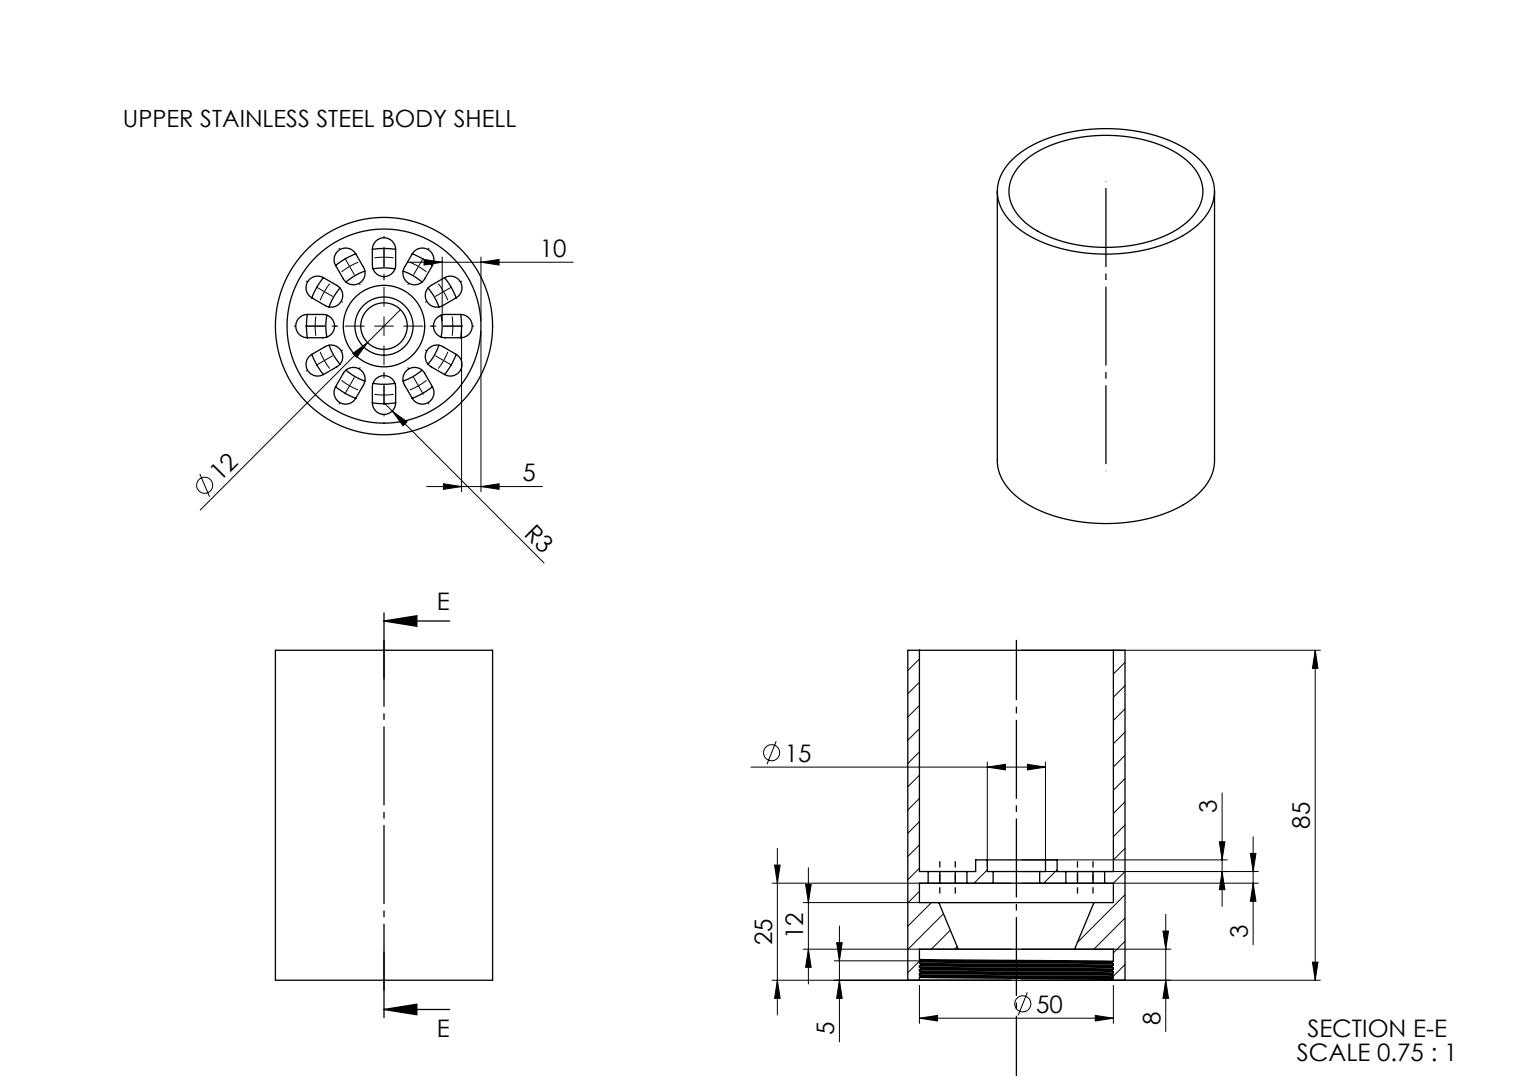
ISO-10303-21;
HEADER;
FILE_DESCRIPTION (('STEP AP214'),
    '1' );
FILE_NAME ('Upper Stainless Steel Body Shell.step',
    '2026-10-04T07:23:31',
    ( '' ),
    ( '' ),
    'SwSTEP 2.0',
    'SolidWorks 2026',
    '' );
FILE_SCHEMA (( 'AUTOMOTIVE_DESIGN' ));
ENDSEC;

DATA;
#1=ORIENTED_EDGE ( 'NONE', *, *, #1320, .F. ) ;
#4=ORIENTED_EDGE ( 'NONE', *, *, #9160, .T. ) ;
#5=AXIS2_PLACEMENT_3D ( 'NONE', #6946, #2717, #1088 ) ;
#6=DIRECTION ( 'NONE',  ( -0.000000000000000000, -1.000000000000000000, -0.000000000000000000 ) ) ;
#9=CARTESIAN_POINT ( 'NONE',  ( 1.507608415688466075E-15, 0.6437499990440845865, -24.62111388750000174 ) ) ;
#11=CARTESIAN_POINT ( 'NONE',  ( -18.60400172474273361, 25.00000000000000000, -7.276923788646512570 ) ) ;
#19=AXIS2_PLACEMENT_3D ( 'NONE', #2994, #5611, #7166 ) ;
#24=CIRCLE ( 'NONE', #8496, 7.500000000000000888 ) ;
#28=ADVANCED_FACE ( 'NONE', ( #7832 ), #3504, .F. ) ;
#29=( BOUNDED_CURVE ( )  B_SPLINE_CURVE ( 2, ( #1490, #9059, #4872, #2466, #7337, #5796, #6516, #4977, #5693, #9821, #8329, #10667, #710, #4147, #8268, #1536, #6469, #7289, #10712, #8217, #9874, #10767, #4922, #6628, #4037, #7506, #659, #2414, #7388, #6572, #5852, #9934, #4089, #2367, #5744, #10884, #9103, #7444, #3285, #9986, #9157, #6688, #4816, #10043, #9208, #3929, #1653, #8998, #5036, #8384, #2255, #5638, #1426, #9505, #8609, #7675, #9449, #6799, #7559, #10941, #4194, #1937, #2745, #104, #163, #6090, #1057, #8554, #946, #4431, #10334, #6920, #2627, #4366, #9319, #6026, #8495, #6851, #10273, #882, #2520 ),
 .UNSPECIFIED., .F., .F. ) 
 B_SPLINE_CURVE_WITH_KNOTS ( ( 3, 2, 2, 2, 2, 2, 2, 2, 2, 2, 2, 2, 2, 2, 2, 2, 2, 2, 2, 2, 2, 2, 2, 2, 2, 2, 2, 2, 2, 2, 2, 2, 2, 2, 2, 2, 2, 2, 2, 2, 3 ),
 ( 0.000000000000000000, 0.02500000000000000139, 0.05000000000000000278, 0.07499999999999999722, 0.1000000000000000056, 0.1250000000000000000, 0.1499999999999999944, 0.1749999999999999889, 0.2000000000000000111, 0.2250000000000000056, 0.2500000000000000000, 0.2750000000000000222, 0.2999999999999999889, 0.3250000000000000111, 0.3499999999999999778, 0.3750000000000000000, 0.4000000000000000222, 0.4249999999999999889, 0.4500000000000000111, 0.4749999999999999778, 0.5000000000000000000, 0.5250000000000000222, 0.5500000000000000444, 0.5749999999999999556, 0.5999999999999999778, 0.6250000000000000000, 0.6500000000000000222, 0.6750000000000000444, 0.6999999999999999556, 0.7249999999999999778, 0.7500000000000000000, 0.7750000000000000222, 0.8000000000000000444, 0.8249999999999999556, 0.8499999999999999778, 0.8750000000000000000, 0.9000000000000000222, 0.9250000000000000444, 0.9499999999999999556, 0.9749999999999999778, 1.000000000000000000 ),
 .UNSPECIFIED. ) 
 CURVE ( )  GEOMETRIC_REPRESENTATION_ITEM ( )  RATIONAL_B_SPLINE_CURVE ( ( 1.000000000000000000, 0.9238795325112867385, 1.000000000000000000, 0.9238795325112867385, 1.000000000000000000, 0.9238795325112867385, 1.000000000000000000, 0.9238795325112867385, 1.000000000000000000, 0.9238795325112867385, 1.000000000000000000, 0.9238795325112867385, 1.000000000000000000, 0.9238795325112867385, 1.000000000000000000, 0.9238795325112867385, 1.000000000000000000, 0.9238795325112867385, 1.000000000000000000, 0.9238795325112867385, 1.000000000000000000, 0.9238795325112867385, 1.000000000000000000, 0.9238795325112867385, 1.000000000000000000, 0.9238795325112867385, 1.000000000000000000, 0.9238795325112867385, 1.000000000000000000, 0.9238795325112867385, 1.000000000000000000, 0.9238795325112867385, 1.000000000000000000, 0.9238795325112867385, 1.000000000000000000, 0.9238795325112867385, 1.000000000000000000, 0.9238795325112867385, 1.000000000000000000, 0.9238795325112867385, 1.000000000000000000, 0.9238795325112867385, 1.000000000000000000, 0.9238795325112867385, 1.000000000000000000, 0.9238795325112867385, 1.000000000000000000, 0.9238795325112867385, 1.000000000000000000, 0.9238795325112867385, 1.000000000000000000, 0.9238795325112867385, 1.000000000000000000, 0.9238795325112867385, 1.000000000000000000, 0.9238795325112867385, 1.000000000000000000, 0.9238795325112867385, 1.000000000000000000, 0.9238795325112867385, 1.000000000000000000, 0.9238795325112867385, 1.000000000000000000, 0.9238795325112867385, 1.000000000000000000, 0.9238795325112867385, 1.000000000000000000, 0.9238795325112867385, 1.000000000000000000, 0.9238795325112867385, 1.000000000000000000, 0.9238795325112867385, 1.000000000000000000, 0.9238795325112867385, 1.000000000000000000, 0.9238795325112867385, 1.000000000000000000, 0.9238795325112867385, 1.000000000000000000, 0.9238795325112867385, 1.000000000000000000 ) ) 
 REPRESENTATION_ITEM ( '' )  );
#35=DIRECTION ( 'NONE',  ( 0.000000000000000000, 0.000000000000000000, 1.000000000000000000 ) ) ;
#36=FACE_OUTER_BOUND ( 'NONE', #8599, .T. ) ;
#38=FACE_OUTER_BOUND ( 'NONE', #4930, .T. ) ;
#40=CIRCLE ( 'NONE', #9387, 2.999999999999999112 ) ;
#46=DIRECTION ( 'NONE',  ( -0.000000000000000000, -1.000000000000000000, -0.000000000000000000 ) ) ;
#55=CARTESIAN_POINT ( 'NONE',  ( 15.13990010960488952, -0.001000000000001000089, -5.276923788646758595 ) ) ;
#56=CARTESIAN_POINT ( 'NONE',  ( 19.74999999999998934, -0.001000000000001000089, -3.000000000000067946 ) ) ;
#58=CARTESIAN_POINT ( 'NONE',  ( -2.999999999999998224, 25.00000000000000000, -15.75000000000000355 ) ) ;
#61=CARTESIAN_POINT ( 'NONE',  ( -4.592425496802574367E-15, 2.362499998088169129, 25.00000000000000000 ) ) ;
#64=VECTOR ( 'NONE', #5356, 1000.000000000000000 ) ;
#65=ORIENTED_EDGE ( 'NONE', *, *, #1287, .F. ) ;
#66=EDGE_CURVE ( 'NONE', #3225, #5856, #203, .T. ) ;
#68=ORIENTED_EDGE ( 'NONE', *, *, #3846, .T. ) ;
#71=DIRECTION ( 'NONE',  ( -0.000000000000000000, -1.000000000000000000, -0.000000000000000000 ) ) ;
#74=CARTESIAN_POINT ( 'NONE',  ( 24.62111388750000174, 2.393749999044084475, 0.000000000000000000 ) ) ;
#75=CARTESIAN_POINT ( 'NONE',  ( -25.00000000000000000, 0.4375000000000000000, -10.35533905932738108 ) ) ;
#76=CARTESIAN_POINT ( 'NONE',  ( 17.10400172474269098, 28.00000000000000000, 9.874999999999957367 ) ) ;
#84=ORIENTED_EDGE ( 'NONE', *, *, #2390, .T. ) ;
#86=DIRECTION ( 'NONE',  ( -0.000000000000000000, 1.000000000000000000, 0.000000000000000000 ) ) ;
#88=FACE_OUTER_BOUND ( 'NONE', #5727, .T. ) ;
#92=CARTESIAN_POINT ( 'NONE',  ( 12.47307621135333200, 25.00000000000000000, 15.60400172474264835 ) ) ;
#93=VERTEX_POINT ( 'NONE', #1861 ) ;
#95=DIRECTION ( 'NONE',  ( -0.000000000000000000, -1.000000000000000000, -0.000000000000000000 ) ) ;
#97=CARTESIAN_POINT ( 'NONE',  ( 24.99999999999999289, 5.549999998088169129, 10.35533905932739529 ) ) ;
#99=ORIENTED_EDGE ( 'NONE', *, *, #3561, .F. ) ;
#101=CARTESIAN_POINT ( 'NONE',  ( 17.10400172474269098, 28.00000000000000000, 9.874999999999957367 ) ) ;
#103=CARTESIAN_POINT ( 'NONE',  ( 19.74999999999998934, 25.00000000000000000, -3.000000000000067946 ) ) ;
#104=CARTESIAN_POINT ( 'NONE',  ( 24.62111388749999108, 4.156249999044084653, 10.19839929293507730 ) ) ;
#106=EDGE_CURVE ( 'NONE', #5745, #5240, #6492, .T. ) ;
#111=ORIENTED_EDGE ( 'NONE', *, *, #6802, .F. ) ;
#112=CARTESIAN_POINT ( 'NONE',  ( 3.061616997868383043E-15, 27.99999999999999645, 25.00000000000000000 ) ) ;
#117=CARTESIAN_POINT ( 'NONE',  ( 2.449293598294706513E-15, 20.00000000000000355, -20.00000000000000000 ) ) ;
#119=EDGE_CURVE ( 'NONE', #6443, #1427, #3381, .T. ) ;
#120=VERTEX_POINT ( 'NONE', #1095 ) ;
#121=ORIENTED_EDGE ( 'NONE', *, *, #10240, .T. ) ;
#122=VERTEX_POINT ( 'NONE', #5243 ) ;
#124=CARTESIAN_POINT ( 'NONE',  ( 0.000000000000000000, 85.00000000000000000, 0.000000000000000000 ) ) ;
#126=CARTESIAN_POINT ( 'NONE',  ( 17.67766952966369232, 0.7374999980881691286, -17.67766952966369232 ) ) ;
#127=CARTESIAN_POINT ( 'NONE',  ( 10.19839929293506486, 1.206249999044084698, 24.62111388749999819 ) ) ;
#128=CARTESIAN_POINT ( 'NONE',  ( -24.62111388750000884, 3.781249999044084653, 10.19839929293505421 ) ) ;
#129=CARTESIAN_POINT ( 'NONE',  ( -25.00000000000001066, 3.174999998088169573, 10.35533905932737397 ) ) ;
#130=EDGE_CURVE ( 'NONE', #7410, #4070, #2608, .T. ) ;
#132=LINE ( 'NONE', #3493, #145 ) ;
#133=FACE_BOUND ( 'NONE', #4065, .T. ) ;
#134=DIRECTION ( 'NONE',  ( 0.000000000000000000, 0.000000000000000000, -1.000000000000000000 ) ) ;
#138=CLOSED_SHELL ( 'NONE', ( #5912, #7027, #10918, #9263, #5268, #8033, #4039, #8931, #9209, #7081, #6514, #516, #6002, #10646, #9653, #6197, #4591, #507, #1397, #6646, #1299, #2039, #10092, #4594, #8749, #861, #6693, #7676, #7148, #10570, #5853, #5516, #7088, #717, #5052, #4023, #6869, #3689, #10249, #2799, #5302, #2691, #9344, #9035, #8964, #1267, #437, #3259, #9811, #1259, #7773, #2191, #3472, #3885, #1656, #6813, #3576, #3914, #8252, #9299, #6399, #2209, #4947, #674, #661, #4449, #10399, #4818, #868, #5935, #9573, #7951, #2937, #7004, #2676, #5317, #5105, #3750, #6202, #28, #5672, #1968, #3916, #4465, #4519, #8455, #4226, #4367, #4978, #6266, #8625, #8205, #7818, #6087, #10928, #4909, #2609 ) ) ;
#139=( BOUNDED_CURVE ( )  B_SPLINE_CURVE ( 2, ( #7817, #6880, #1965, #10238, #251, #129, #4337, #7756, #2653 ),
 .UNSPECIFIED., .F., .F. ) 
 B_SPLINE_CURVE_WITH_KNOTS ( ( 3, 2, 2, 2, 3 ),
 ( 0.4500000000000000111, 0.4749999999999999778, 0.5000000000000000000, 0.5250000000000000222, 0.5500000000000000444 ),
 .UNSPECIFIED. ) 
 CURVE ( )  GEOMETRIC_REPRESENTATION_ITEM ( )  RATIONAL_B_SPLINE_CURVE ( ( 1.000000000000000000, 0.9238795325112867385, 1.000000000000000000, 0.9238795325112867385, 1.000000000000000000, 0.9238795325112867385, 1.000000000000000000, 0.9238795325112867385, 1.000000000000000000 ) ) 
 REPRESENTATION_ITEM ( '' )  );
#140=ORIENTED_EDGE ( 'NONE', *, *, #5576, .T. ) ;
#141=ORIENTED_EDGE ( 'NONE', *, *, #3333, .T. ) ;
#145=VECTOR ( 'NONE', #2655, 1000.000000000000000 ) ;
#147=CARTESIAN_POINT ( 'NONE',  ( -17.10400172474254532, 28.00000000000000000, 9.875000000000202505 ) ) ;
#149=FACE_OUTER_BOUND ( 'NONE', #10908, .T. ) ;
#152=CARTESIAN_POINT ( 'NONE',  ( -24.62111388750000174, 3.893749999044084475, -3.015216831376932151E-15 ) ) ;
#155=ORIENTED_EDGE ( 'NONE', *, *, #4589, .F. ) ;
#156=CARTESIAN_POINT ( 'NONE',  ( 24.99999999999999289, 4.937500000000000888, 10.35533905932739529 ) ) ;
#157=CARTESIAN_POINT ( 'NONE',  ( 17.67766952966368521, 5.487499998088169129, 17.67766952966369232 ) ) ;
#163=CARTESIAN_POINT ( 'NONE',  ( 24.62111388750000174, 4.218749999044084653, 0.000000000000000000 ) ) ;
#168=ORIENTED_EDGE ( 'NONE', *, *, #8555, .T. ) ;
#169=DIRECTION ( 'NONE',  ( -0.000000000000000000, 1.000000000000000000, 0.000000000000000000 ) ) ;
#170=CARTESIAN_POINT ( 'NONE',  ( -17.10400172474254532, 28.00000000000000000, 9.875000000000202505 ) ) ;
#179=EDGE_LOOP ( 'NONE', ( #3319, #1358, #7705, #7107 ) ) ;
#181=ORIENTED_EDGE ( 'NONE', *, *, #2071, .F. ) ;
#186=CARTESIAN_POINT ( 'NONE',  ( -10.35533905932737575, 3.924999998088169129, -25.00000000000000000 ) ) ;
#187=CARTESIAN_POINT ( 'NONE',  ( -17.40975659021752975, 3.593749999044084653, -17.40975659021752975 ) ) ;
#188=FACE_OUTER_BOUND ( 'NONE', #7003, .T. ) ;
#189=AXIS2_PLACEMENT_3D ( 'NONE', #10549, #390, #1123 ) ;
#190=VECTOR ( 'NONE', #6922, 1000.000000000000000 ) ;
#192=PLANE ( 'NONE',  #1400 ) ;
#198=ORIENTED_EDGE ( 'NONE', *, *, #7378, .T. ) ;
#199=ORIENTED_EDGE ( 'NONE', *, *, #10771, .T. ) ;
#201=AXIS2_PLACEMENT_3D ( 'NONE', #9799, #474, #7991 ) ;
#203=LINE ( 'NONE', #6782, #2239 ) ;
#205=DIRECTION ( 'NONE',  ( -0.000000000000000000, 1.000000000000000000, -0.000000000000000000 ) ) ;
#208=CARTESIAN_POINT ( 'NONE',  ( -3.223142256880076948E-15, 28.00000000000000000, -15.75000000000000000 ) ) ;
#209=DIRECTION ( 'NONE',  ( 0.000000000000000000, 0.000000000000000000, 1.000000000000000000 ) ) ;
#210=CARTESIAN_POINT ( 'NONE',  ( 7.874999999999916511, 28.00000000000000000, -10.63990010960495702 ) ) ;
#211=CARTESIAN_POINT ( 'NONE',  ( 1.530808498934191521E-15, 1.250000000000000000, -25.00000000000000000 ) ) ;
#212=AXIS2_PLACEMENT_3D ( 'NONE', #8810, #4790, #575 ) ;
#214=ORIENTED_EDGE ( 'NONE', *, *, #10048, .F. ) ;
#215=DIRECTION ( 'NONE',  ( 0.000000000000000000, 0.000000000000000000, 1.000000000000000000 ) ) ;
#216=CARTESIAN_POINT ( 'NONE',  ( -10.35533905932739174, 4.299999998088169129, 24.99999999999999289 ) ) ;
#217=CIRCLE ( 'NONE', #6933, 25.00000000000000000 ) ;
#220=CARTESIAN_POINT ( 'NONE',  ( 3.061616997868383043E-15, 0.000000000000000000, 25.00000000000000000 ) ) ;
#225=AXIS2_PLACEMENT_3D ( 'NONE', #3856, #484, #9861 ) ;
#229=VECTOR ( 'NONE', #2900, 1000.000000000000000 ) ;
#230=CARTESIAN_POINT ( 'NONE',  ( 24.99999999999999289, 1.937500000000000000, 10.35533905932739529 ) ) ;
#231=CARTESIAN_POINT ( 'NONE',  ( -4.522825247065398226E-15, 4.968749999044083765, 24.62111388750000174 ) ) ;
#233=ORIENTED_EDGE ( 'NONE', *, *, #10324, .F. ) ;
#234=CARTESIAN_POINT ( 'NONE',  ( 1.530808498934191521E-15, 0.8624999980881691286, -25.00000000000000000 ) ) ;
#235=CARTESIAN_POINT ( 'NONE',  ( -17.67766952966368876, 2.375000000000000000, -17.67766952966369232 ) ) ;
#238=DIRECTION ( 'NONE',  ( -0.000000000000000000, 1.000000000000000000, -0.000000000000000000 ) ) ;
#239=VECTOR ( 'NONE', #5384, 1000.000000000000000 ) ;
#241=VERTEX_POINT ( 'NONE', #8761 ) ;
#247=EDGE_CURVE ( 'NONE', #3577, #5793, #9294, .T. ) ;
#248=CARTESIAN_POINT ( 'NONE',  ( -25.00000000000001421, 3.174999998088169129, 10.35533905932737397 ) ) ;
#249=CARTESIAN_POINT ( 'NONE',  ( -24.62111388750000174, 2.656249999044085097, -10.19839929293506131 ) ) ;
#251=CARTESIAN_POINT ( 'NONE',  ( -25.00000000000000000, 3.112499998088169129, -3.061616997868383043E-15 ) ) ;
#252=CYLINDRICAL_SURFACE ( 'NONE', #1418, 25.00000000000000000 ) ;
#255=CARTESIAN_POINT ( 'NONE',  ( -13.63990010960498367, 28.00000000000000000, -4.874999999999871214 ) ) ;
#258=VECTOR ( 'NONE', #8917, 1000.000000000000114 ) ;
#261=EDGE_CURVE ( 'NONE', #5968, #10806, #9690, .T. ) ;
#264=DIRECTION ( 'NONE',  ( 0.000000000000000000, 0.000000000000000000, 1.000000000000000000 ) ) ;
#269=CARTESIAN_POINT ( 'NONE',  ( -17.40975659021752975, 3.768749999044084475, -17.40975659021752975 ) ) ;
#284=CARTESIAN_POINT ( 'NONE',  ( 10.35533905932737930, 3.187500000000000444, -25.00000000000000000 ) ) ;
#285=CARTESIAN_POINT ( 'NONE',  ( -10.19839929293505776, 0.7062499990440845865, -24.62111388750000174 ) ) ;
#288=CARTESIAN_POINT ( 'NONE',  ( 1.530808498934191521E-15, 2.250000000000000444, -25.00000000000000000 ) ) ;
#297=DIRECTION ( 'NONE',  ( -2.168404344971010347E-16, 0.000000000000000000, -1.000000000000000000 ) ) ;
#298=CARTESIAN_POINT ( 'NONE',  ( 10.35533905932737930, 2.799999998088169573, -25.00000000000000000 ) ) ;
#299=CARTESIAN_POINT ( 'NONE',  ( 24.62111388749999463, 4.156249999044083765, 10.19839929293507730 ) ) ;
#300=CYLINDRICAL_SURFACE ( 'NONE', #10201, 2.999999999999997335 ) ;
#304=CARTESIAN_POINT ( 'NONE',  ( -15.75000000000000000, 25.00000000000000000, 1.681956355172181189E-13 ) ) ;
#305=ORIENTED_EDGE ( 'NONE', *, *, #6800, .T. ) ;
#306=ORIENTED_EDGE ( 'NONE', *, *, #2066, .F. ) ;
#311=LINE ( 'NONE', #7774, #4484 ) ;
#313=CARTESIAN_POINT ( 'NONE',  ( 0.000000000000000000, 0.000000000000000000, 0.000000000000000000 ) ) ;
#315=CYLINDRICAL_SURFACE ( 'NONE', #5866, 2.999999999999997335 ) ;
#316=CARTESIAN_POINT ( 'NONE',  ( 17.40975659021752975, 3.518749999044084920, -17.40975659021752975 ) ) ;
#321=ORIENTED_EDGE ( 'NONE', *, *, #1197, .F. ) ;
#323=EDGE_CURVE ( 'NONE', #8872, #4838, #1231, .T. ) ;
#326=FACE_OUTER_BOUND ( 'NONE', #1511, .T. ) ;
#329=CARTESIAN_POINT ( 'NONE',  ( -10.35533905932735621, 5.299999998088170905, 25.00000000000003197 ) ) ;
#331=AXIS2_PLACEMENT_3D ( 'NONE', #9569, #2055, #5387 ) ;
#333=ORIENTED_EDGE ( 'NONE', *, *, #7900, .F. ) ;
#335=EDGE_CURVE ( 'NONE', #6402, #2102, #10397, .T. ) ;
#339=LINE ( 'NONE', #8784, #5857 ) ;
#345=CARTESIAN_POINT ( 'NONE',  ( 2.999999999999999112, -0.001000000000001000089, 19.75000000000000000 ) ) ;
#350=CARTESIAN_POINT ( 'NONE',  ( -17.40975659021753330, 5.018749999044084475, 17.40975659021752975 ) ) ;
#351=CARTESIAN_POINT ( 'NONE',  ( 17.67766952966368521, 4.875000000000000000, 17.67766952966369232 ) ) ;
#360=ORIENTED_EDGE ( 'NONE', *, *, #10700, .T. ) ;
#368=CARTESIAN_POINT ( 'NONE',  ( 15.60400172474260927, -0.001000000000001000089, -12.47307621135339062 ) ) ;
#372=CIRCLE ( 'NONE', #6199, 2.999999999999999112 ) ;
#380=CYLINDRICAL_SURFACE ( 'NONE', #9214, 2.999999999999997335 ) ;
#389=AXIS2_PLACEMENT_3D ( 'NONE', #6634, #9992, #10835 ) ;
#390=DIRECTION ( 'NONE',  ( 0.000000000000000000, 0.000000000000000000, 1.000000000000000000 ) ) ;
#392=CARTESIAN_POINT ( 'NONE',  ( 15.60400172474269453, 25.00000000000000000, 12.47307621135327693 ) ) ;
#395=LINE ( 'NONE', #6422, #1735 ) ;
#398=EDGE_CURVE ( 'NONE', #963, #2292, #395, .T. ) ;
#400=EDGE_LOOP ( 'NONE', ( #8892, #7575 ) ) ;
#402=CIRCLE ( 'NONE', #9394, 2.999999999999999112 ) ;
#406=CARTESIAN_POINT ( 'NONE',  ( 24.62111388750000174, 2.393749999044084475, 0.000000000000000000 ) ) ;
#407=CARTESIAN_POINT ( 'NONE',  ( -25.00000000000000000, 3.437500000000000000, -10.35533905932738108 ) ) ;
#410=CARTESIAN_POINT ( 'NONE',  ( -17.67766952966368876, 0.9874999980881691286, -17.67766952966369232 ) ) ;
#412=AXIS2_PLACEMENT_3D ( 'NONE', #4846, #684, #4789 ) ;
#414=EDGE_CURVE ( 'NONE', #5784, #652, #8731, .T. ) ;
#416=VERTEX_POINT ( 'NONE', #5429 ) ;
#418=ORIENTED_EDGE ( 'NONE', *, *, #7281, .F. ) ;
#419=ORIENTED_EDGE ( 'NONE', *, *, #8806, .F. ) ;
#424=FACE_OUTER_BOUND ( 'NONE', #721, .T. ) ;
#433=DIRECTION ( 'NONE',  ( 1.000000000000000000, 0.000000000000000000, 0.000000000000000000 ) ) ;
#436=EDGE_CURVE ( 'NONE', #1816, #8189, #1374, .T. ) ;
#437=ADVANCED_FACE ( 'NONE', ( #450 ), #10554, .F. ) ;
#439=EDGE_CURVE ( 'NONE', #3209, #9663, #8791, .T. ) ;
#441=CARTESIAN_POINT ( 'NONE',  ( -4.592425496802574367E-15, 5.362499998088169129, 25.00000000000000000 ) ) ;
#442=CARTESIAN_POINT ( 'NONE',  ( 1.507608415688466075E-15, 2.643749999044084920, -24.62111388750000174 ) ) ;
#444=CARTESIAN_POINT ( 'NONE',  ( 24.62111388750000174, 5.218749999044084653, 0.000000000000000000 ) ) ;
#448=VERTEX_POINT ( 'NONE', #1591 ) ;
#450=FACE_OUTER_BOUND ( 'NONE', #4386, .T. ) ;
#451=PRODUCT ( 'Upper Stainless Steel Body Shell', 'Upper Stainless Steel Body Shell', '', ( #5141 ) ) ;
#452=ORIENTED_EDGE ( 'NONE', *, *, #7524, .T. ) ;
#456=CARTESIAN_POINT ( 'NONE',  ( -17.40975659021752975, 1.768749999044084475, -17.40975659021752975 ) ) ;
#458=CARTESIAN_POINT ( 'NONE',  ( -25.00000000000000000, 1.437500000000000000, -10.35533905932738108 ) ) ;
#459=EDGE_CURVE ( 'NONE', #2069, #3931, #29, .T. ) ;
#461=DIRECTION ( 'NONE',  ( 0.000000000000000000, -0.000000000000000000, 1.000000000000000000 ) ) ;
#463=CARTESIAN_POINT ( 'NONE',  ( 17.67766952966369232, 3.737499998088169573, -17.67766952966369232 ) ) ;
#464=ORIENTED_EDGE ( 'NONE', *, *, #335, .T. ) ;
#465=ORIENTED_EDGE ( 'NONE', *, *, #1592, .F. ) ;
#469=EDGE_CURVE ( 'NONE', #8735, #3294, #3407, .T. ) ;
#471=EDGE_LOOP ( 'NONE', ( #8532, #9181, #9575, #7189, #4997, #4095, #6051, #9424 ) ) ;
#474=DIRECTION ( 'NONE',  ( 0.000000000000000000, 1.000000000000000000, 0.000000000000000000 ) ) ;
#475=DIRECTION ( 'NONE',  ( 0.000000000000000000, 0.000000000000000000, 1.000000000000000000 ) ) ;
#476=ORIENTED_EDGE ( 'NONE', *, *, #10844, .F. ) ;
#483=DIRECTION ( 'NONE',  ( 0.000000000000000000, 1.000000000000000000, 0.000000000000000000 ) ) ;
#484=DIRECTION ( 'NONE',  ( -0.8660254037844451469, 0.000000000000000000, -0.4999999999999887312 ) ) ;
#486=VECTOR ( 'NONE', #920, 1000.000000000000000 ) ;
#489=CARTESIAN_POINT ( 'NONE',  ( 19.75000000000001066, 28.00000000000000000, 2.999999999999927613 ) ) ;
#493=DIRECTION ( 'NONE',  ( -0.000000000000000000, -1.000000000000000000, -0.000000000000000000 ) ) ;
#497=AXIS2_PLACEMENT_3D ( 'NONE', #5910, #6978, #9384 ) ;
#500=VERTEX_POINT ( 'NONE', #5316 ) ;
#504=CARTESIAN_POINT ( 'NONE',  ( 24.62111388749999463, 2.331249999044084031, 10.19839929293507730 ) ) ;
#506=CARTESIAN_POINT ( 'NONE',  ( 25.00000000000000000, 4.062500000000000000, -10.35533905932737753 ) ) ;
#507=ADVANCED_FACE ( 'NONE', ( #3586 ), #10212, .F. ) ;
#508=EDGE_CURVE ( 'NONE', #3100, #1857, #9259, .T. ) ;
#509=DIRECTION ( 'NONE',  ( -0.000000000000000000, -1.000000000000000000, -0.000000000000000000 ) ) ;
#510=CARTESIAN_POINT ( 'NONE',  ( 25.00000000000000000, 0.6749999980881690176, -10.35533905932737753 ) ) ;
#511=DIRECTION ( 'NONE',  ( 0.000000000000000000, 0.000000000000000000, 1.000000000000000000 ) ) ;
#513=ORIENTED_EDGE ( 'NONE', *, *, #1407, .T. ) ;
#516=ADVANCED_FACE ( 'NONE', ( #8437 ), #4251, .F. ) ;
#518=LINE ( 'NONE', #3202, #8425 ) ;
#520=EDGE_CURVE ( 'NONE', #5481, #3253, #2570, .T. ) ;
#522=DIRECTION ( 'NONE',  ( -0.000000000000000000, 1.000000000000000000, -0.000000000000000000 ) ) ;
#527=CIRCLE ( 'NONE', #8986, 2.999999999999998668 ) ;
#534=VECTOR ( 'NONE', #1707, 1000.000000000000000 ) ;
#538=EDGE_LOOP ( 'NONE', ( #10942, #1687, #7523, #476 ) ) ;
#539=VECTOR ( 'NONE', #2027, 1000.000000000000000 ) ;
#543=CARTESIAN_POINT ( 'NONE',  ( 10.19839929293505953, 3.581249999044085364, -24.62111388750000174 ) ) ;
#545=CARTESIAN_POINT ( 'NONE',  ( 19.75000000000000000, -0.001000000000001000089, -7.291468677852036884E-14 ) ) ;
#548=DIRECTION ( 'NONE',  ( -0.000000000000000000, 1.000000000000000000, -0.000000000000000000 ) ) ;
#551=VECTOR ( 'NONE', #10567, 1000.000000000000000 ) ;
#554=CARTESIAN_POINT ( 'NONE',  ( -24.62111388750000174, 3.893749999044084475, -3.015216831376932151E-15 ) ) ;
#555=CARTESIAN_POINT ( 'NONE',  ( -4.592425496802574367E-15, 4.750000000000000000, 25.00000000000000000 ) ) ;
#556=VECTOR ( 'NONE', #169, 1000.000000000000000 ) ;
#558=CARTESIAN_POINT ( 'NONE',  ( -13.63990010960481492, 28.00000000000000000, 7.875000000000163425 ) ) ;
#562=ORIENTED_EDGE ( 'NONE', *, *, #9891, .F. ) ;
#565=AXIS2_PLACEMENT_3D ( 'NONE', #8099, #5732, #433 ) ;
#571=( NAMED_UNIT ( * ) PLANE_ANGLE_UNIT ( ) SI_UNIT ( $, .RADIAN. ) );
#572=AXIS2_PLACEMENT_3D ( 'NONE', #5272, #10857, #4120 ) ;
#575=DIRECTION ( 'NONE',  ( 0.000000000000000000, 0.000000000000000000, -1.000000000000000000 ) ) ;
#577=CARTESIAN_POINT ( 'NONE',  ( -15.60400172474251690, 28.00000000000000000, 12.47307621135349720 ) ) ;
#580=ORIENTED_EDGE ( 'NONE', *, *, #5350, .F. ) ;
#582=EDGE_LOOP ( 'NONE', ( #4342, #8954, #2146, #5276, #930 ) ) ;
#584=ORIENTED_EDGE ( 'NONE', *, *, #5586, .F. ) ;
#598=LINE ( 'NONE', #3011, #2601 ) ;
#601=CARTESIAN_POINT ( 'NONE',  ( -24.62111388750000884, 2.956249999044084475, 10.19839929293505421 ) ) ;
#607=EDGE_LOOP ( 'NONE', ( #9268, #5348, #7147, #5082, #6374 ) ) ;
#608=ORIENTED_EDGE ( 'NONE', *, *, #5350, .T. ) ;
#611=CARTESIAN_POINT ( 'NONE',  ( 24.62111388750000174, 5.393749999044085364, 0.000000000000000000 ) ) ;
#612=EDGE_LOOP ( 'NONE', ( #729, #7297, #168, #8289 ) ) ;
#614=( BOUNDED_CURVE ( )  B_SPLINE_CURVE ( 2, ( #3089, #1344, #5599, #8078, #6437, #9838, #463, #1440, #10520 ),
 .UNSPECIFIED., .F., .F. ) 
 B_SPLINE_CURVE_WITH_KNOTS ( ( 3, 2, 2, 2, 3 ),
 ( 0.5500000000000000444, 0.5749999999999999556, 0.5999999999999999778, 0.6250000000000000000, 0.6500000000000000222 ),
 .UNSPECIFIED. ) 
 CURVE ( )  GEOMETRIC_REPRESENTATION_ITEM ( )  RATIONAL_B_SPLINE_CURVE ( ( 1.000000000000000000, 0.9238795325112867385, 1.000000000000000000, 0.9238795325112867385, 1.000000000000000000, 0.9238795325112867385, 1.000000000000000000, 0.9238795325112867385, 1.000000000000000000 ) ) 
 REPRESENTATION_ITEM ( '' )  );
#616=CARTESIAN_POINT ( 'NONE',  ( 25.00000000000000000, 1.674999998088169351, -10.35533905932737753 ) ) ;
#621=ORIENTED_EDGE ( 'NONE', *, *, #1452, .F. ) ;
#624=CARTESIAN_POINT ( 'NONE',  ( -10.19839929293505776, 0.5312499990440845421, -24.62111388750000174 ) ) ;
#633=ORIENTED_EDGE ( 'NONE', *, *, #8885, .F. ) ;
#634=VERTEX_POINT ( 'NONE', #10183 ) ;
#635=ORIENTED_EDGE ( 'NONE', *, *, #6976, .T. ) ;
#636=EDGE_CURVE ( 'NONE', #9541, #9951, #1793, .T. ) ;
#637=EDGE_LOOP ( 'NONE', ( #10358, #10252, #5332, #5163 ) ) ;
#640=CARTESIAN_POINT ( 'NONE',  ( -2.999999999999996447, 25.00000000000000000, 19.75000000000000000 ) ) ;
#641=EDGE_CURVE ( 'NONE', #2931, #7240, #5287, .T. ) ;
#642=CARTESIAN_POINT ( 'NONE',  ( 17.67766952966368521, 3.875000000000000000, 17.67766952966369232 ) ) ;
#644=CARTESIAN_POINT ( 'NONE',  ( -12.13990010960501031, -0.001000000000001000089, -10.47307621135320410 ) ) ;
#646=EDGE_CURVE ( 'NONE', #6058, #5812, #132, .T. ) ;
#651=CARTESIAN_POINT ( 'NONE',  ( 24.62111388750000174, 3.456249999044084920, -10.19839929293505776 ) ) ;
#652=VERTEX_POINT ( 'NONE', #1852 ) ;
#655=DIRECTION ( 'NONE',  ( -0.000000000000000000, -1.000000000000000000, -0.000000000000000000 ) ) ;
#659=CARTESIAN_POINT ( 'NONE',  ( -17.40975659021753330, 1.843749999044084653, 17.40975659021752975 ) ) ;
#661=ADVANCED_FACE ( 'NONE', ( #7154 ), #8753, .F. ) ;
#665=CARTESIAN_POINT ( 'NONE',  ( 10.19839929293506486, 1.031249999044084653, 24.62111388749999819 ) ) ;
#668=CARTESIAN_POINT ( 'NONE',  ( -7.875000000000116351, -0.001000000000001000089, -13.63990010960484334 ) ) ;
#669=LINE ( 'NONE', #7401, #7772 ) ;
#674=ADVANCED_FACE ( 'NONE', ( #2881 ), #5596, .F. ) ;
#675=CIRCLE ( 'NONE', #6169, 15.00000000000000178 ) ;
#678=ORIENTED_EDGE ( 'NONE', *, *, #6885, .F. ) ;
#679=ORIENTED_EDGE ( 'NONE', *, *, #641, .F. ) ;
#681=CARTESIAN_POINT ( 'NONE',  ( -4.522825247065398226E-15, 0.9687499990440845421, 24.62111388750000174 ) ) ;
#682=DIRECTION ( 'NONE',  ( 0.8660254037844399289, 0.000000000000000000, 0.4999999999999978351 ) ) ;
#683=CARTESIAN_POINT ( 'NONE',  ( -18.60400172474257730, 25.00000000000000000, 7.276923788646904256 ) ) ;
#684=DIRECTION ( 'NONE',  ( 0.000000000000000000, 1.000000000000000000, 0.000000000000000000 ) ) ;
#690=ORIENTED_EDGE ( 'NONE', *, *, #10232, .T. ) ;
#695=DIRECTION ( 'NONE',  ( 0.000000000000000000, 0.000000000000000000, -1.000000000000000000 ) ) ;
#696=AXIS2_PLACEMENT_3D ( 'NONE', #5366, #10629, #1398 ) ;
#697=VECTOR ( 'NONE', #9069, 1000.000000000000000 ) ;
#700=AXIS2_PLACEMENT_3D ( 'NONE', #7174, #7076, #7125 ) ;
#703=AXIS2_PLACEMENT_3D ( 'NONE', #3703, #2954, #6358 ) ;
#710=CARTESIAN_POINT ( 'NONE',  ( -4.522825247065398226E-15, 0.9687499990440845421, 24.62111388750000174 ) ) ;
#712=ORIENTED_EDGE ( 'NONE', *, *, #4302, .T. ) ;
#713=VECTOR ( 'NONE', #2272, 1000.000000000000000 ) ;
#714=ORIENTED_EDGE ( 'NONE', *, *, #5386, .T. ) ;
#715=ADVANCED_BREP_SHAPE_REPRESENTATION ( '', ( #10733, #7040 ), #6327 ) ;
#716=VERTEX_POINT ( 'NONE', #6382 ) ;
#717=ADVANCED_FACE ( 'NONE', ( #1386 ), #8129, .T. ) ;
#720=CARTESIAN_POINT ( 'NONE',  ( -10.19839929293505776, 3.531249999044084653, -24.62111388750000174 ) ) ;
#721=EDGE_LOOP ( 'NONE', ( #2374, #8932, #8644, #8469 ) ) ;
#722=CARTESIAN_POINT ( 'NONE',  ( 15.13990010960488952, 28.00000000000000000, -5.276923788646758595 ) ) ;
#728=VECTOR ( 'NONE', #9849, 1000.000000000000000 ) ;
#729=ORIENTED_EDGE ( 'NONE', *, *, #3055, .T. ) ;
#730=ORIENTED_EDGE ( 'NONE', *, *, #9628, .F. ) ;
#734=VECTOR ( 'NONE', #3164, 999.9999999999998863 ) ;
#735=CARTESIAN_POINT ( 'NONE',  ( 24.62111388749999463, 3.331249999044084920, 10.19839929293507730 ) ) ;
#736=DIRECTION ( 'NONE',  ( 0.000000000000000000, 0.000000000000000000, 1.000000000000000000 ) ) ;
#741=FACE_BOUND ( 'NONE', #6305, .T. ) ;
#745=ORIENTED_EDGE ( 'NONE', *, *, #6957, .T. ) ;
#746=CIRCLE ( 'NONE', #6240, 2.999999999999999112 ) ;
#750=EDGE_LOOP ( 'NONE', ( #8386, #3432 ) ) ;
#751=VECTOR ( 'NONE', #9383, 1000.000000000000000 ) ;
#752=VECTOR ( 'NONE', #4466, 1000.000000000000000 ) ;
#755=FACE_OUTER_BOUND ( 'NONE', #919, .T. ) ;
#767=ORIENTED_EDGE ( 'NONE', *, *, #8949, .F. ) ;
#778=EDGE_CURVE ( 'NONE', #2292, #917, #6434, .T. ) ;
#780=DIRECTION ( 'NONE',  ( -0.000000000000000000, 1.000000000000000000, -0.000000000000000000 ) ) ;
#781=CARTESIAN_POINT ( 'NONE',  ( 24.62111388750000174, 1.218749999044084431, 0.000000000000000000 ) ) ;
#783=ORIENTED_EDGE ( 'NONE', *, *, #7325, .T. ) ;
#788=LINE ( 'NONE', #4206, #9032 ) ;
#790=CARTESIAN_POINT ( 'NONE',  ( -12.47307621135311351, 28.00000000000000000, 15.60400172474282599 ) ) ;
#792=EDGE_CURVE ( 'NONE', #3303, #9988, #3484, .T. ) ;
#794=EDGE_LOOP ( 'NONE', ( #9614, #452, #10633, #7368 ) ) ;
#798=CARTESIAN_POINT ( 'NONE',  ( 24.62111388750000174, 3.393749999044084475, 0.000000000000000000 ) ) ;
#799=CARTESIAN_POINT ( 'NONE',  ( 17.40975659021752975, 1.343749999044084653, -17.40975659021752975 ) ) ;
#802=FACE_BOUND ( 'NONE', #1466, .T. ) ;
#803=DIRECTION ( 'NONE',  ( -0.4999999999999886757, 0.000000000000000000, 0.8660254037844452579 ) ) ;
#807=ORIENTED_EDGE ( 'NONE', *, *, #2469, .F. ) ;
#809=ORIENTED_EDGE ( 'NONE', *, *, #4102, .F. ) ;
#814=DIRECTION ( 'NONE',  ( 0.8660254037844344888, 0.000000000000000000, -0.5000000000000074385 ) ) ;
#815=CARTESIAN_POINT ( 'NONE',  ( 0.000000000000000000, 85.00000000000000000, -25.00000000000000000 ) ) ;
#822=CYLINDRICAL_SURFACE ( 'NONE', #4192, 5.999999999999999112 ) ;
#831=DIRECTION ( 'NONE',  ( -3.469446951953617344E-15, 0.000000000000000000, 1.000000000000000000 ) ) ;
#832=CARTESIAN_POINT ( 'NONE',  ( -17.40975659021753330, 0.8437499990440846531, 17.40975659021752975 ) ) ;
#833=FACE_OUTER_BOUND ( 'NONE', #9928, .T. ) ;
#835=DIRECTION ( 'NONE',  ( 0.000000000000000000, 1.000000000000000000, -0.000000000000000000 ) ) ;
#837=CARTESIAN_POINT ( 'NONE',  ( -15.75000000000003553, -0.001000000000001000089, -2.999999999999832578 ) ) ;
#841=ORIENTED_EDGE ( 'NONE', *, *, #5114, .F. ) ;
#843=LINE ( 'NONE', #1077, #3128 ) ;
#846=CARTESIAN_POINT ( 'NONE',  ( -24.62111388750000174, 1.893749999044084475, -3.015216831376932151E-15 ) ) ;
#847=CARTESIAN_POINT ( 'NONE',  ( 17.40975659021752620, 2.093749999044084653, 17.40975659021753330 ) ) ;
#848=VECTOR ( 'NONE', #6164, 1000.000000000000000 ) ;
#849=VERTEX_POINT ( 'NONE', #3356 ) ;
#852=VECTOR ( 'NONE', #9676, 1000.000000000000000 ) ;
#855=EDGE_CURVE ( 'NONE', #3253, #7713, #7400, .T. ) ;
#857=VERTEX_POINT ( 'NONE', #5867 ) ;
#861=ADVANCED_FACE ( 'NONE', ( #10783 ), #9999, .F. ) ;
#864=CARTESIAN_POINT ( 'NONE',  ( 10.47307621135333200, -0.001000000000001000089, 12.13990010960489840 ) ) ;
#867=DIRECTION ( 'NONE',  ( -0.000000000000000000, -1.000000000000000000, -0.000000000000000000 ) ) ;
#868=ADVANCED_FACE ( 'NONE', ( #9887 ), #9068, .F. ) ;
#876=PLANE ( 'NONE',  #6905 ) ;
#879=AXIS2_PLACEMENT_3D ( 'NONE', #8342, #7460, #2375 ) ;
#881=DIRECTION ( 'NONE',  ( 0.000000000000000000, 1.000000000000000000, 0.000000000000000000 ) ) ;
#882=CARTESIAN_POINT ( 'NONE',  ( 24.62111388749999108, 5.156249999044084653, 10.19839929293507730 ) ) ;
#883=VERTEX_POINT ( 'NONE', #5047 ) ;
#884=AXIS2_PLACEMENT_3D ( 'NONE', #2622, #6916, #2566 ) ;
#888=DIRECTION ( 'NONE',  ( -0.000000000000000000, -1.000000000000000000, -0.000000000000000000 ) ) ;
#890=DIRECTION ( 'NONE',  ( -0.5000000000000073275, 0.000000000000000000, -0.8660254037844343777 ) ) ;
#891=ORIENTED_EDGE ( 'NONE', *, *, #4982, .F. ) ;
#892=DIRECTION ( 'NONE',  ( -1.734723475976808672E-15, 0.000000000000000000, 1.000000000000000000 ) ) ;
#896=DIRECTION ( 'NONE',  ( -0.000000000000000000, -1.000000000000000000, -0.000000000000000000 ) ) ;
#900=ORIENTED_EDGE ( 'NONE', *, *, #1135, .T. ) ;
#901=EDGE_LOOP ( 'NONE', ( #712, #6645, #5603, #3659 ) ) ;
#902=ORIENTED_EDGE ( 'NONE', *, *, #7656, .F. ) ;
#905=LINE ( 'NONE', #10177, #2160 ) ;
#906=CARTESIAN_POINT ( 'NONE',  ( -24.62111388750000174, 1.831249999044084475, -10.19839929293506131 ) ) ;
#907=CARTESIAN_POINT ( 'NONE',  ( 24.99999999999999289, 0.9374999999999998890, 10.35533905932739529 ) ) ;
#916=EDGE_CURVE ( 'NONE', #4798, #3364, #4990, .T. ) ;
#917=VERTEX_POINT ( 'NONE', #7517 ) ;
#918=AXIS2_PLACEMENT_3D ( 'NONE', #5764, #9129, #6604 ) ;
#919=EDGE_LOOP ( 'NONE', ( #68, #2381, #5556, #7537 ) ) ;
#920=DIRECTION ( 'NONE',  ( 0.000000000000000000, 1.000000000000000000, -0.000000000000000000 ) ) ;
#921=EDGE_CURVE ( 'NONE', #8104, #9229, #2426, .T. ) ;
#923=ORIENTED_EDGE ( 'NONE', *, *, #1153, .F. ) ;
#927=DIRECTION ( 'NONE',  ( -0.8660254037844402619, -0.4999999999999971134, 0.000000000000000000 ) ) ;
#928=DIRECTION ( 'NONE',  ( -0.000000000000000000, 1.000000000000000000, -0.000000000000000000 ) ) ;
#930=ORIENTED_EDGE ( 'NONE', *, *, #5640, .F. ) ;
#931=EDGE_CURVE ( 'NONE', #3835, #5793, #3995, .T. ) ;
#932=AXIS2_PLACEMENT_3D ( 'NONE', #8431, #1760, #6794 ) ;
#933=CIRCLE ( 'NONE', #6057, 2.999999999999997335 ) ;
#935=VECTOR ( 'NONE', #8204, 1000.000000000000000 ) ;
#936=EDGE_CURVE ( 'NONE', #10359, #5295, #2788, .T. ) ;
#939=DIRECTION ( 'NONE',  ( 0.000000000000000000, 0.000000000000000000, 1.000000000000000000 ) ) ;
#940=AXIS2_PLACEMENT_3D ( 'NONE', #6069, #10195, #10363 ) ;
#941=CARTESIAN_POINT ( 'NONE',  ( -15.60400172474278158, 28.00000000000000000, -12.47307621135316680 ) ) ;
#946=CARTESIAN_POINT ( 'NONE',  ( 1.507608415688466075E-15, 4.468749999044084653, -24.62111388750000174 ) ) ;
#952=CARTESIAN_POINT ( 'NONE',  ( 17.67766952966368521, 1.875000000000000000, 17.67766952966369232 ) ) ;
#953=AXIS2_PLACEMENT_3D ( 'NONE', #6193, #7077, #10436 ) ;
#954=CARTESIAN_POINT ( 'NONE',  ( 10.19839929293506486, 5.031249999044083765, 24.62111388749999819 ) ) ;
#961=CARTESIAN_POINT ( 'NONE',  ( 0.000000000000000000, 28.00000000000000000, -7.500000000000000888 ) ) ;
#963=VERTEX_POINT ( 'NONE', #10056 ) ;
#965=EDGE_LOOP ( 'NONE', ( #9121, #8922, #199, #5165 ) ) ;
#966=ORIENTED_EDGE ( 'NONE', *, *, #8610, .T. ) ;
#968=CARTESIAN_POINT ( 'NONE',  ( 3.957930336368489021E-15, 28.00000000000000000, 19.75000000000000000 ) ) ;
#970=CARTESIAN_POINT ( 'NONE',  ( 1.507608415688466075E-15, 0.6437499990440845865, -24.62111388750000174 ) ) ;
#971=CARTESIAN_POINT ( 'NONE',  ( 17.40975659021752620, 1.268749999044084475, 17.40975659021753330 ) ) ;
#972=CARTESIAN_POINT ( 'NONE',  ( -24.62111388750000884, 2.781249999044085541, 10.19839929293505421 ) ) ;
#974=FACE_BOUND ( 'NONE', #8390, .T. ) ;
#975=CYLINDRICAL_SURFACE ( 'NONE', #2480, 25.00000000000000000 ) ;
#976=LINE ( 'NONE', #2030, #752 ) ;
#980=DIRECTION ( 'NONE',  ( 0.000000000000000000, -1.000000000000000000, 0.000000000000000000 ) ) ;
#981=ORIENTED_EDGE ( 'NONE', *, *, #5799, .F. ) ;
#983=CARTESIAN_POINT ( 'NONE',  ( 0.000000000000000000, 20.00000000000000355, 20.00000000000000000 ) ) ;
#989=ORIENTED_EDGE ( 'NONE', *, *, #1979, .F. ) ;
#993=CARTESIAN_POINT ( 'NONE',  ( -10.35533905932737575, 3.924999998088168685, -25.00000000000000000 ) ) ;
#994=EDGE_CURVE ( 'NONE', #9664, #5784, #7058, .T. ) ;
#998=DIRECTION ( 'NONE',  ( 0.5000000000000009992, 0.000000000000000000, 0.8660254037844380415 ) ) ;
#1005=CARTESIAN_POINT ( 'NONE',  ( 25.00000000000000000, 3.062500000000000000, -10.35533905932737753 ) ) ;
#1006=DIRECTION ( 'NONE',  ( 0.000000000000000000, 1.000000000000000000, 0.000000000000000000 ) ) ;
#1009=DIRECTION ( 'NONE',  ( -0.8660254037844328234, 0.000000000000000000, 0.5000000000000098810 ) ) ;
#1011=DIRECTION ( 'NONE',  ( -0.4999999999999888978, 0.000000000000000000, 0.8660254037844450359 ) ) ;
#1012=FACE_BOUND ( 'NONE', #6871, .T. ) ;
#1014=DIRECTION ( 'NONE',  ( -0.000000000000000000, 1.000000000000000000, -0.000000000000000000 ) ) ;
#1018=EDGE_LOOP ( 'NONE', ( #3836, #1523 ) ) ;
#1020=CARTESIAN_POINT ( 'NONE',  ( 9.184850993605149917E-16, 31.00000000000000000, 7.500000000000000888 ) ) ;
#1023=CARTESIAN_POINT ( 'NONE',  ( 17.67766952966369232, 4.737499998088169129, -17.67766952966369232 ) ) ;
#1024=CARTESIAN_POINT ( 'NONE',  ( -17.40975659021753330, 4.843749999044083765, 17.40975659021752975 ) ) ;
#1028=FACE_OUTER_BOUND ( 'NONE', #4958, .T. ) ;
#1029=STYLED_ITEM ( 'NONE', ( #4490 ), #10733 ) ;
#1033=EDGE_LOOP ( 'NONE', ( #9297, #6954, #9499, #8643 ) ) ;
#1034=ORIENTED_EDGE ( 'NONE', *, *, #10874, .F. ) ;
#1036=( GEOMETRIC_REPRESENTATION_CONTEXT ( 3 ) GLOBAL_UNCERTAINTY_ASSIGNED_CONTEXT ( ( #3144 ) ) GLOBAL_UNIT_ASSIGNED_CONTEXT ( ( #2061, #10617, #3724 ) ) REPRESENTATION_CONTEXT ( 'NONE', 'WORKASPACE' ) );
#1038=PLANE ( 'NONE',  #2001 ) ;
#1040=DIRECTION ( 'NONE',  ( -0.000000000000000000, -1.000000000000000000, -0.000000000000000000 ) ) ;
#1042=CARTESIAN_POINT ( 'NONE',  ( -7.875000000000116351, 25.00000000000000000, -13.63990010960484334 ) ) ;
#1044=FACE_OUTER_BOUND ( 'NONE', #8271, .T. ) ;
#1046=APPLICATION_CONTEXT ( 'automotive_design' ) ;
#1050=CARTESIAN_POINT ( 'NONE',  ( -4.592425496802574367E-15, 5.362499998088169129, 25.00000000000000000 ) ) ;
#1052=( BOUNDED_CURVE ( )  B_SPLINE_CURVE ( 2, ( #2193, #5570, #7270, #10650, #3059, #6455, #2236, #1412, #4073 ),
 .UNSPECIFIED., .F., .F. ) 
 B_SPLINE_CURVE_WITH_KNOTS ( ( 3, 2, 2, 2, 3 ),
 ( 0.7500000000000000000, 0.7750000000000000222, 0.8000000000000000444, 0.8250000000000000666, 0.8500000000000000888 ),
 .UNSPECIFIED. ) 
 CURVE ( )  GEOMETRIC_REPRESENTATION_ITEM ( )  RATIONAL_B_SPLINE_CURVE ( ( 1.000000000000000000, 0.9238795325112867385, 1.000000000000000000, 0.9238795325112867385, 1.000000000000000000, 0.9238795325112867385, 1.000000000000000000, 0.9238795325112864054, 1.000000000000000444 ) ) 
 REPRESENTATION_ITEM ( '' )  );
#1053=LINE ( 'NONE', #4308, #3154 ) ;
#1057=CARTESIAN_POINT ( 'NONE',  ( 17.40975659021752975, 4.343749999044084653, -17.40975659021752975 ) ) ;
#1064=VERTEX_POINT ( 'NONE', #4444 ) ;
#1065=FACE_OUTER_BOUND ( 'NONE', #3101, .T. ) ;
#1066=EDGE_CURVE ( 'NONE', #241, #6044, #675, .T. ) ;
#1075=EDGE_CURVE ( 'NONE', #9988, #3378, #10729, .T. ) ;
#1076=ORIENTED_EDGE ( 'NONE', *, *, #4297, .F. ) ;
#1077=CARTESIAN_POINT ( 'NONE',  ( -15.74999999999997158, -0.001000000000001000089, 3.000000000000165645 ) ) ;
#1080=CARTESIAN_POINT ( 'NONE',  ( -25.00000000000001421, 4.174999998088169129, 10.35533905932737397 ) ) ;
#1081=CARTESIAN_POINT ( 'NONE',  ( -24.62111388750000884, 4.781249999044083765, 10.19839929293505421 ) ) ;
#1086=DIRECTION ( 'NONE',  ( 0.000000000000000000, -1.000000000000000000, 0.000000000000000000 ) ) ;
#1087=LINE ( 'NONE', #7821, #4265 ) ;
#1088=DIRECTION ( 'NONE',  ( 0.000000000000000000, 0.000000000000000000, 1.000000000000000000 ) ) ;
#1095=CARTESIAN_POINT ( 'NONE',  ( 2.999999999999997335, 28.00000000000000000, -15.75000000000000355 ) ) ;
#1098=CARTESIAN_POINT ( 'NONE',  ( -4.592425496802574367E-15, 2.750000000000000000, 25.00000000000000000 ) ) ;
#1099=FACE_OUTER_BOUND ( 'NONE', #4676, .T. ) ;
#1100=DIRECTION ( 'NONE',  ( -0.000000000000000000, -1.000000000000000000, -0.000000000000000000 ) ) ;
#1103=CARTESIAN_POINT ( 'NONE',  ( 24.62111388749999463, 4.331249999044084475, 10.19839929293507730 ) ) ;
#1106=ORIENTED_EDGE ( 'NONE', *, *, #4297, .T. ) ;
#1114=CARTESIAN_POINT ( 'NONE',  ( 0.000000000000000000, 85.00000000000000000, -25.00000000000000000 ) ) ;
#1118=AXIS2_PLACEMENT_3D ( 'NONE', #8201, #3910, #5621 ) ;
#1119=FACE_OUTER_BOUND ( 'NONE', #5894, .T. ) ;
#1121=DIRECTION ( 'NONE',  ( 0.000000000000000000, 1.000000000000000000, -0.000000000000000000 ) ) ;
#1123=DIRECTION ( 'NONE',  ( 1.000000000000000000, 0.000000000000000000, -0.000000000000000000 ) ) ;
#1130=ORIENTED_EDGE ( 'NONE', *, *, #1287, .T. ) ;
#1131=CIRCLE ( 'NONE', #9596, 25.00000000000000000 ) ;
#1132=ORIENTED_EDGE ( 'NONE', *, *, #9956, .T. ) ;
#1135=EDGE_CURVE ( 'NONE', #6439, #7005, #598, .T. ) ;
#1139=CARTESIAN_POINT ( 'NONE',  ( 25.00000000000000000, 0.6749999980881691286, -10.35533905932737753 ) ) ;
#1140=CARTESIAN_POINT ( 'NONE',  ( 10.35533905932738286, 3.424999998088169573, 24.99999999999999645 ) ) ;
#1142=CARTESIAN_POINT ( 'NONE',  ( 24.62111388750000174, 4.218749999044084653, 0.000000000000000000 ) ) ;
#1144=EDGE_CURVE ( 'NONE', #4659, #9481, #7929, .T. ) ;
#1150=AXIS2_PLACEMENT_3D ( 'NONE', #9805, #4699, #8881 ) ;
#1152=DIRECTION ( 'NONE',  ( 0.000000000000000000, 0.000000000000000000, -1.000000000000000000 ) ) ;
#1153=EDGE_CURVE ( 'NONE', #7275, #5714, #1385, .T. ) ;
#1157=EDGE_CURVE ( 'NONE', #7830, #2468, #8435, .T. ) ;
#1162=CARTESIAN_POINT ( 'NONE',  ( -25.00000000000000000, 1.500000000000000000, -3.061616997868383043E-15 ) ) ;
#1163=DIRECTION ( 'NONE',  ( 0.000000000000000000, 0.000000000000000000, 1.000000000000000000 ) ) ;
#1165=ORIENTED_EDGE ( 'NONE', *, *, #6990, .F. ) ;
#1170=DIRECTION ( 'NONE',  ( -0.000000000000000000, -1.000000000000000000, -0.000000000000000000 ) ) ;
#1173=ORIENTED_EDGE ( 'NONE', *, *, #4852, .F. ) ;
#1180=CARTESIAN_POINT ( 'NONE',  ( 0.000000000000000000, 85.00000000000000000, -28.00000000000000000 ) ) ;
#1182=DIRECTION ( 'NONE',  ( 0.5000000000000073275, 0.000000000000000000, 0.8660254037844343777 ) ) ;
#1187=CARTESIAN_POINT ( 'NONE',  ( 17.40975659021752975, 4.518749999044085364, -17.40975659021752975 ) ) ;
#1188=CARTESIAN_POINT ( 'NONE',  ( -25.00000000000000000, 4.112499998088169129, -3.061616997868383043E-15 ) ) ;
#1189=CARTESIAN_POINT ( 'NONE',  ( -17.67766952966369232, 3.625000000000000000, 17.67766952966368876 ) ) ;
#1190=CARTESIAN_POINT ( 'NONE',  ( 25.00000000000000000, 8.000000000000003553, 0.000000000000000000 ) ) ;
#1193=DIRECTION ( 'NONE',  ( -0.8660254037844362651, 0.000000000000000000, 0.5000000000000042188 ) ) ;
#1194=LINE ( 'NONE', #8583, #1830 ) ;
#1195=ORIENTED_EDGE ( 'NONE', *, *, #9439, .F. ) ;
#1197=EDGE_CURVE ( 'NONE', #9938, #6120, #10204, .T. ) ;
#1202=DIRECTION ( 'NONE',  ( 0.000000000000000000, 0.000000000000000000, 1.000000000000000000 ) ) ;
#1204=CARTESIAN_POINT ( 'NONE',  ( 17.10400172474269098, 25.00000000000000000, 9.874999999999957367 ) ) ;
#1205=AXIS2_PLACEMENT_3D ( 'NONE', #2985, #7162, #9742 ) ;
#1208=CARTESIAN_POINT ( 'NONE',  ( -10.19839929293505776, 3.706249999044084920, -24.62111388750000174 ) ) ;
#1209=AXIS2_PLACEMENT_3D ( 'NONE', #6734, #5206, #8547 ) ;
#1212=AXIS2_PLACEMENT_3D ( 'NONE', #668, #8227, #10723 ) ;
#1215=CARTESIAN_POINT ( 'NONE',  ( 0.000000000000000000, 85.00000000000000000, 0.000000000000000000 ) ) ;
#1217=DIRECTION ( 'NONE',  ( 0.000000000000000000, 0.000000000000000000, -1.000000000000000000 ) ) ;
#1219=DIRECTION ( 'NONE',  ( 0.000000000000000000, 1.000000000000000000, -0.000000000000000000 ) ) ;
#1225=CARTESIAN_POINT ( 'NONE',  ( 17.40975659021752975, 0.5187499990440845865, -17.40975659021752975 ) ) ;
#1227=VERTEX_POINT ( 'NONE', #5840 ) ;
#1231=LINE ( 'NONE', #7145, #1714 ) ;
#1236=CARTESIAN_POINT ( 'NONE',  ( -17.40975659021752975, 4.768749999044085364, -17.40975659021752975 ) ) ;
#1237=CARTESIAN_POINT ( 'NONE',  ( -4.592425496802574367E-15, 3.750000000000000000, 25.00000000000000000 ) ) ;
#1242=VECTOR ( 'NONE', #4786, 999.9999999999998863 ) ;
#1250=DIRECTION ( 'NONE',  ( 0.000000000000000000, 1.000000000000000000, 0.000000000000000000 ) ) ;
#1255=LINE ( 'NONE', #2784, #3930 ) ;
#1259=ADVANCED_FACE ( 'NONE', ( #5878 ), #9404, .F. ) ;
#1265=CIRCLE ( 'NONE', #212, 2.999999999999999112 ) ;
#1267=ADVANCED_FACE ( 'NONE', ( #9340 ), #5228, .F. ) ;
#1276=CARTESIAN_POINT ( 'NONE',  ( 10.19839929293506486, 5.206249999044084475, 24.62111388749999819 ) ) ;
#1277=ORIENTED_EDGE ( 'NONE', *, *, #2943, .F. ) ;
#1284=ORIENTED_EDGE ( 'NONE', *, *, #6471, .T. ) ;
#1287=EDGE_CURVE ( 'NONE', #3078, #448, #6936, .T. ) ;
#1292=CARTESIAN_POINT ( 'NONE',  ( -10.19839929293507552, 4.081249999044084475, 24.62111388749999463 ) ) ;
#1294=CARTESIAN_POINT ( 'NONE',  ( 15.13990010960488952, 25.00000000000000000, -5.276923788646758595 ) ) ;
#1297=CARTESIAN_POINT ( 'NONE',  ( -10.35533905932737575, 0.9249999980881692396, -25.00000000000000000 ) ) ;
#1299=ADVANCED_FACE ( 'NONE', ( #3543 ), #3366, .F. ) ;
#1303=CIRCLE ( 'NONE', #4668, 2.999999999999997335 ) ;
#1305=VECTOR ( 'NONE', #8382, 1000.000000000000000 ) ;
#1307=DIRECTION ( 'NONE',  ( -0.000000000000000000, 1.000000000000000000, -0.000000000000000000 ) ) ;
#1308=CARTESIAN_POINT ( 'NONE',  ( 1.285879139104720831E-15, 31.00000000000000000, 10.50000000000000000 ) ) ;
#1309=CARTESIAN_POINT ( 'NONE',  ( -7.276923788646840308, -0.001000000000001000089, -18.60400172474260216 ) ) ;
#1310=DIRECTION ( 'NONE',  ( 2.168404344971010594E-16, 0.000000000000000000, 1.000000000000000000 ) ) ;
#1311=CIRCLE ( 'NONE', #412, 10.50000000000000000 ) ;
#1313=CARTESIAN_POINT ( 'NONE',  ( 0.000000000000000000, 85.00000000000000000, 0.000000000000000000 ) ) ;
#1314=DIRECTION ( 'NONE',  ( 0.000000000000000000, 0.000000000000000000, -1.000000000000000000 ) ) ;
#1317=CARTESIAN_POINT ( 'NONE',  ( -19.75000000000003197, 25.00000000000000000, -2.999999999999789946 ) ) ;
#1320=EDGE_CURVE ( 'NONE', #10806, #10642, #2710, .T. ) ;
#1324=CARTESIAN_POINT ( 'NONE',  ( 12.47307621135322186, 28.00000000000000000, -15.60400172474273717 ) ) ;
#1325=CARTESIAN_POINT ( 'NONE',  ( 17.40975659021752975, 4.518749999044084475, -17.40975659021752975 ) ) ;
#1331=EDGE_CURVE ( 'NONE', #716, #8104, #5972, .T. ) ;
#1334=VERTEX_POINT ( 'NONE', #1020 ) ;
#1335=ORIENTED_EDGE ( 'NONE', *, *, #5586, .T. ) ;
#1336=EDGE_CURVE ( 'NONE', #6439, #3577, #843, .T. ) ;
#1337=CARTESIAN_POINT ( 'NONE',  ( -2.999999999999999112, 28.00000000000000000, -19.75000000000000000 ) ) ;
#1339=CARTESIAN_POINT ( 'NONE',  ( 24.62111388750000174, 3.456249999044084920, -10.19839929293505776 ) ) ;
#1340=CARTESIAN_POINT ( 'NONE',  ( 10.35533905932738286, 2.812500000000000000, 24.99999999999999645 ) ) ;
#1342=CARTESIAN_POINT ( 'NONE',  ( -25.00000000000000000, 2.049999998088169129, -10.35533905932738108 ) ) ;
#1343=CARTESIAN_POINT ( 'NONE',  ( 0.000000000000000000, 25.00000000000000000, 0.000000000000000000 ) ) ;
#1344=CARTESIAN_POINT ( 'NONE',  ( 10.35533905932738286, 3.424999998088169129, 24.99999999999999645 ) ) ;
#1347=ORIENTED_EDGE ( 'NONE', *, *, #414, .T. ) ;
#1348=ORIENTED_EDGE ( 'NONE', *, *, #1803, .T. ) ;
#1350=CARTESIAN_POINT ( 'NONE',  ( -10.35533905932735621, 4.687500000000000888, 25.00000000000003197 ) ) ;
#1352=LINE ( 'NONE', #2121, #5707 ) ;
#1353=CARTESIAN_POINT ( 'NONE',  ( -9.874999999999777955, 28.00000000000000000, 20.10400172474279401 ) ) ;
#1358=ORIENTED_EDGE ( 'NONE', *, *, #9661, .T. ) ;
#1363=CARTESIAN_POINT ( 'NONE',  ( -4.592425496802574367E-15, 3.750000000000000000, 25.00000000000000000 ) ) ;
#1370=CARTESIAN_POINT ( 'NONE',  ( -10.19839929293507375, 5.081249999044084475, 24.62111388749999108 ) ) ;
#1374=CIRCLE ( 'NONE', #1916, 20.00000000000000000 ) ;
#1376=CARTESIAN_POINT ( 'NONE',  ( 17.67766952966369232, 2.737499998088169573, -17.67766952966369232 ) ) ;
#1383=CARTESIAN_POINT ( 'NONE',  ( -24.62111388750000174, 3.831249999044084920, -10.19839929293506131 ) ) ;
#1384=CARTESIAN_POINT ( 'NONE',  ( -17.67766952966369232, 4.625000000000000000, 17.67766952966368876 ) ) ;
#1385=( BOUNDED_CURVE ( )  B_SPLINE_CURVE ( 2, ( #7665, #9200, #3274, #156, #10089 ),
 .UNSPECIFIED., .F., .F. ) 
 B_SPLINE_CURVE_WITH_KNOTS ( ( 3, 2, 3 ),
 ( 0.9500000000000000666, 0.9750000000000000888, 1.000000000000000000 ),
 .UNSPECIFIED. ) 
 CURVE ( )  GEOMETRIC_REPRESENTATION_ITEM ( )  RATIONAL_B_SPLINE_CURVE ( ( 0.9999999999999996669, 0.9238795325112870716, 1.000000000000000000, 0.9238795325112867385, 1.000000000000000000 ) ) 
 REPRESENTATION_ITEM ( '' )  );
#1386=FACE_OUTER_BOUND ( 'NONE', #3015, .T. ) ;
#1387=DIRECTION ( 'NONE',  ( 0.000000000000000000, 1.000000000000000000, 0.000000000000000000 ) ) ;
#1390=EDGE_CURVE ( 'NONE', #9703, #8735, #3858, .T. ) ;
#1391=ORIENTED_EDGE ( 'NONE', *, *, #1336, .F. ) ;
#1397=ADVANCED_FACE ( 'NONE', ( #3603 ), #1785, .F. ) ;
#1398=DIRECTION ( 'NONE',  ( 1.000000000000000000, 0.000000000000000000, 0.000000000000000000 ) ) ;
#1400=AXIS2_PLACEMENT_3D ( 'NONE', #7820, #2766, #461 ) ;
#1404=DIRECTION ( 'NONE',  ( -0.000000000000000000, 1.000000000000000000, -0.000000000000000000 ) ) ;
#1407=EDGE_CURVE ( 'NONE', #4897, #9663, #7369, .T. ) ;
#1408=ORIENTED_EDGE ( 'NONE', *, *, #7379, .F. ) ;
#1411=DIRECTION ( 'NONE',  ( -0.000000000000000000, 1.000000000000000000, -0.000000000000000000 ) ) ;
#1412=CARTESIAN_POINT ( 'NONE',  ( 10.35533905932734733, 4.799999998088170905, -25.00000000000004263 ) ) ;
#1416=CARTESIAN_POINT ( 'NONE',  ( 2.999999999999997335, -0.001000000000001000089, -15.75000000000000355 ) ) ;
#1418=AXIS2_PLACEMENT_3D ( 'NONE', #6999, #2218, #3946 ) ;
#1421=CARTESIAN_POINT ( 'NONE',  ( -24.62111388750000174, 2.893749999044084475, -3.015216831376932151E-15 ) ) ;
#1422=VERTEX_POINT ( 'NONE', #1337 ) ;
#1426=CARTESIAN_POINT ( 'NONE',  ( 1.507608415688466075E-15, 3.468749999044085097, -24.62111388750000174 ) ) ;
#1427=VERTEX_POINT ( 'NONE', #4516 ) ;
#1429=VERTEX_POINT ( 'NONE', #2875 ) ;
#1431=DIRECTION ( 'NONE',  ( 0.000000000000000000, 1.000000000000000000, 0.000000000000000000 ) ) ;
#1432=CARTESIAN_POINT ( 'NONE',  ( 24.62111388750000174, 3.218749999044084653, 0.000000000000000000 ) ) ;
#1436=CIRCLE ( 'NONE', #6396, 2.999999999999999112 ) ;
#1437=CARTESIAN_POINT ( 'NONE',  ( -17.67766952966368876, 1.987499998088169129, -17.67766952966369232 ) ) ;
#1438=CARTESIAN_POINT ( 'NONE',  ( 10.35533905932738286, 1.424999998088169129, 24.99999999999999645 ) ) ;
#1440=CARTESIAN_POINT ( 'NONE',  ( 10.35533905932737930, 3.799999998088170461, -25.00000000000000000 ) ) ;
#1441=AXIS2_PLACEMENT_3D ( 'NONE', #9150, #10878, #939 ) ;
#1452=EDGE_CURVE ( 'NONE', #10359, #9337, #5390, .T. ) ;
#1457=AXIS2_PLACEMENT_3D ( 'NONE', #1881, #4430, #2626 ) ;
#1458=EDGE_LOOP ( 'NONE', ( #10032, #6332, #5618, #10903 ) ) ;
#1461=CIRCLE ( 'NONE', #3767, 2.999999999999999112 ) ;
#1466=EDGE_LOOP ( 'NONE', ( #9188, #419, #9134, #2277, #8530 ) ) ;
#1467=ORIENTED_EDGE ( 'NONE', *, *, #6471, .F. ) ;
#1470=VECTOR ( 'NONE', #9381, 1000.000000000000000 ) ;
#1476=CARTESIAN_POINT ( 'NONE',  ( -12.13990010960478827, 28.00000000000000000, 10.47307621135345990 ) ) ;
#1479=CIRCLE ( 'NONE', #8350, 2.999999999999996891 ) ;
#1481=CARTESIAN_POINT ( 'NONE',  ( 12.47307621135322186, -0.001000000000001000089, -15.60400172474273717 ) ) ;
#1483=CARTESIAN_POINT ( 'NONE',  ( -10.19839929293507375, 2.081249999044084920, 24.62111388749999108 ) ) ;
#1485=CYLINDRICAL_SURFACE ( 'NONE', #4776, 2.999999999999997780 ) ;
#1489=CARTESIAN_POINT ( 'NONE',  ( 18.60400172474263414, 28.00000000000000000, -7.276923788646775471 ) ) ;
#1490=CARTESIAN_POINT ( 'NONE',  ( 24.62111388750000174, 0.2187499990440845699, 0.000000000000000000 ) ) ;
#1491=ORIENTED_EDGE ( 'NONE', *, *, #636, .T. ) ;
#1496=CARTESIAN_POINT ( 'NONE',  ( -17.40975659021753330, 3.843749999044085097, 17.40975659021752975 ) ) ;
#1501=LINE ( 'NONE', #1717, #5855 ) ;
#1503=ORIENTED_EDGE ( 'NONE', *, *, #6130, .T. ) ;
#1511=EDGE_LOOP ( 'NONE', ( #9359, #9062, #8305, #4763 ) ) ;
#1513=VERTEX_POINT ( 'NONE', #7872 ) ;
#1523=ORIENTED_EDGE ( 'NONE', *, *, #3552, .T. ) ;
#1525=EDGE_CURVE ( 'NONE', #2067, #3638, #5542, .T. ) ;
#1529=ORIENTED_EDGE ( 'NONE', *, *, #414, .F. ) ;
#1532=CARTESIAN_POINT ( 'NONE',  ( -12.47307621135344391, 25.00000000000000000, -15.60400172474256131 ) ) ;
#1533=ORIENTED_EDGE ( 'NONE', *, *, #1752, .F. ) ;
#1534=VECTOR ( 'NONE', #4374, 1000.000000000000000 ) ;
#1536=CARTESIAN_POINT ( 'NONE',  ( 24.62111388749999108, 1.156249999044084431, 10.19839929293507730 ) ) ;
#1538=ORIENTED_EDGE ( 'NONE', *, *, #4642, .F. ) ;
#1540=COLOUR_RGB ( '', 0.09019608, 0.27058824, 0.51372549) ;
#1541=EDGE_CURVE ( 'NONE', #3501, #5714, #9841, .T. ) ;
#1545=CARTESIAN_POINT ( 'NONE',  ( 17.40975659021752620, 3.093749999044084653, 17.40975659021753330 ) ) ;
#1547=PLANE ( 'NONE',  #1764 ) ;
#1549=DIRECTION ( 'NONE',  ( -0.4999999999999947820, 0.000000000000000000, 0.8660254037844417052 ) ) ;
#1550=DIRECTION ( 'NONE',  ( 0.000000000000000000, 0.000000000000000000, -1.000000000000000000 ) ) ;
#1555=AXIS2_PLACEMENT_3D ( 'NONE', #3516, #95, #35 ) ;
#1558=CARTESIAN_POINT ( 'NONE',  ( 10.19839929293506486, 2.031249999044084653, 24.62111388749999819 ) ) ;
#1559=CARTESIAN_POINT ( 'NONE',  ( -12.13990010960478827, 25.00000000000000000, 10.47307621135345634 ) ) ;
#1566=ORIENTED_EDGE ( 'NONE', *, *, #5716, .F. ) ;
#1567=VERTEX_POINT ( 'NONE', #5711 ) ;
#1569=FACE_OUTER_BOUND ( 'NONE', #3975, .T. ) ;
#1573=CARTESIAN_POINT ( 'NONE',  ( 25.00000000000000000, 4.062500000000000000, -10.35533905932737753 ) ) ;
#1575=VECTOR ( 'NONE', #3300, 1000.000000000000000 ) ;
#1576=EDGE_CURVE ( 'NONE', #1567, #10596, #8541, .T. ) ;
#1580=LINE ( 'NONE', #9867, #4734 ) ;
#1590=CARTESIAN_POINT ( 'NONE',  ( 2.999999999999996447, 28.00000000000000000, -19.75000000000000000 ) ) ;
#1591=CARTESIAN_POINT ( 'NONE',  ( -2.999999999999997335, 28.00000000000000000, 15.75000000000000355 ) ) ;
#1592=EDGE_CURVE ( 'NONE', #6402, #10131, #6909, .T. ) ;
#1594=ORIENTED_EDGE ( 'NONE', *, *, #4781, .F. ) ;
#1598=CARTESIAN_POINT ( 'NONE',  ( 7.276923788646575630, 28.00000000000000000, -18.60400172474270519 ) ) ;
#1599=CARTESIAN_POINT ( 'NONE',  ( 17.40975659021752620, 2.093749999044084653, 17.40975659021753330 ) ) ;
#1600=CARTESIAN_POINT ( 'NONE',  ( 17.10400172474261637, -0.001000000000001000089, -9.875000000000085265 ) ) ;
#1604=CARTESIAN_POINT ( 'NONE',  ( 19.74999999999998934, 28.00000000000000000, -3.000000000000067946 ) ) ;
#1608=CIRCLE ( 'NONE', #19, 28.00000000000000000 ) ;
#1613=ORIENTED_EDGE ( 'NONE', *, *, #855, .F. ) ;
#1615=ORIENTED_EDGE ( 'NONE', *, *, #3849, .F. ) ;
#1617=CARTESIAN_POINT ( 'NONE',  ( 10.19839929293505953, 0.4062499990440845421, -24.62111388750000174 ) ) ;
#1622=DIRECTION ( 'NONE',  ( -0.000000000000000000, -1.000000000000000000, -0.000000000000000000 ) ) ;
#1623=EDGE_CURVE ( 'NONE', #10846, #3100, #2615, .T. ) ;
#1629=EDGE_LOOP ( 'NONE', ( #7601, #1408 ) ) ;
#1641=CIRCLE ( 'NONE', #4499, 2.999999999999998224 ) ;
#1645=DIRECTION ( 'NONE',  ( 0.000000000000000000, 0.000000000000000000, 1.000000000000000000 ) ) ;
#1651=CIRCLE ( 'NONE', #1150, 7.500000000000000888 ) ;
#1653=CARTESIAN_POINT ( 'NONE',  ( 17.40975659021752620, 3.093749999044084653, 17.40975659021753330 ) ) ;
#1656=ADVANCED_FACE ( 'NONE', ( #5950 ), #9433, .F. ) ;
#1661=CARTESIAN_POINT ( 'NONE',  ( 10.19839929293506486, 5.206249999044084475, 24.62111388749999819 ) ) ;
#1669=DIRECTION ( 'NONE',  ( 0.000000000000000000, 1.000000000000000000, 0.000000000000000000 ) ) ;
#1671=VERTEX_POINT ( 'NONE', #5196 ) ;
#1673=VERTEX_POINT ( 'NONE', #210 ) ;
#1675=DIRECTION ( 'NONE',  ( -0.000000000000000000, -1.000000000000000000, -0.000000000000000000 ) ) ;
#1676=EDGE_CURVE ( 'NONE', #7970, #10189, #9176, .T. ) ;
#1677=CARTESIAN_POINT ( 'NONE',  ( 24.62111388750000174, 3.456249999044084920, -10.19839929293505776 ) ) ;
#1678=CARTESIAN_POINT ( 'NONE',  ( -17.40975659021753330, 1.843749999044084653, 17.40975659021752975 ) ) ;
#1682=CARTESIAN_POINT ( 'NONE',  ( -7.874999999999821476, 28.00000000000000000, 13.63990010960501031 ) ) ;
#1684=LINE ( 'NONE', #9355, #8514 ) ;
#1685=EDGE_LOOP ( 'NONE', ( #2047, #6952, #2247, #8218 ) ) ;
#1687=ORIENTED_EDGE ( 'NONE', *, *, #1197, .T. ) ;
#1690=DIRECTION ( 'NONE',  ( 0.000000000000000000, 0.000000000000000000, -1.000000000000000000 ) ) ;
#1692=DIRECTION ( 'NONE',  ( -0.000000000000000000, 1.000000000000000000, 0.000000000000000000 ) ) ;
#1695=VERTEX_POINT ( 'NONE', #10321 ) ;
#1696=EDGE_CURVE ( 'NONE', #3821, #2862, #3161, .T. ) ;
#1701=DIRECTION ( 'NONE',  ( -0.000000000000000000, -1.000000000000000000, -0.000000000000000000 ) ) ;
#1703=CARTESIAN_POINT ( 'NONE',  ( -17.67766952966369232, 5.237499998088169129, 17.67766952966368876 ) ) ;
#1704=DIRECTION ( 'NONE',  ( -0.000000000000000000, 1.000000000000000000, -0.000000000000000000 ) ) ;
#1707=DIRECTION ( 'NONE',  ( -0.8660254037844361541, 0.000000000000000000, 0.5000000000000042188 ) ) ;
#1708=CARTESIAN_POINT ( 'NONE',  ( -10.19839929293507552, 3.906249999044085097, 24.62111388749999463 ) ) ;
#1709=DIRECTION ( 'NONE',  ( -1.000000000000000000, 0.000000000000000000, 3.708321773340234242E-15 ) ) ;
#1714=VECTOR ( 'NONE', #1182, 1000.000000000000114 ) ;
#1715=EDGE_CURVE ( 'NONE', #6058, #7041, #5359, .T. ) ;
#1717=CARTESIAN_POINT ( 'NONE',  ( 0.000000000000000000, 85.00000000000000000, -25.00000000000000000 ) ) ;
#1729=CARTESIAN_POINT ( 'NONE',  ( 10.35533905932738286, 0.8125000000000001110, 24.99999999999999645 ) ) ;
#1732=EDGE_CURVE ( 'NONE', #9229, #2686, #4962, .T. ) ;
#1734=CARTESIAN_POINT ( 'NONE',  ( -15.60400172474278158, 25.00000000000000000, -12.47307621135316680 ) ) ;
#1735=VECTOR ( 'NONE', #5585, 1000.000000000000000 ) ;
#1737=CARTESIAN_POINT ( 'NONE',  ( -19.75000000000003197, 25.00000000000000000, -2.999999999999789946 ) ) ;
#1748=( BOUNDED_CURVE ( )  B_SPLINE_CURVE ( 2, ( #6391, #9845, #10685, #3838, #4731, #3043, #5608, #1350, #8725 ),
 .UNSPECIFIED., .F., .F. ) 
 B_SPLINE_CURVE_WITH_KNOTS ( ( 3, 2, 2, 2, 3 ),
 ( 0.8500000000000000888, 0.8750000000000001110, 0.9000000000000001332, 0.9250000000000001554, 0.9500000000000000666 ),
 .UNSPECIFIED. ) 
 CURVE ( )  GEOMETRIC_REPRESENTATION_ITEM ( )  RATIONAL_B_SPLINE_CURVE ( ( 0.9999999999999996669, 0.9238795325112870716, 1.000000000000000000, 0.9238795325112867385, 1.000000000000000000, 0.9238795325112867385, 1.000000000000000000, 0.9238795325112864054, 1.000000000000000444 ) ) 
 REPRESENTATION_ITEM ( '' )  );
#1749=DIRECTION ( 'NONE',  ( -0.000000000000000000, 1.000000000000000000, -0.000000000000000000 ) ) ;
#1750=DIRECTION ( 'NONE',  ( -0.000000000000000000, -1.000000000000000000, -0.000000000000000000 ) ) ;
#1752=EDGE_CURVE ( 'NONE', #2032, #917, #8974, .T. ) ;
#1753=ORIENTED_EDGE ( 'NONE', *, *, #6602, .F. ) ;
#1754=CARTESIAN_POINT ( 'NONE',  ( 1.530808498934191521E-15, 1.862499998088169129, -25.00000000000000000 ) ) ;
#1760=DIRECTION ( 'NONE',  ( 0.000000000000000000, 1.000000000000000000, 0.000000000000000000 ) ) ;
#1761=PLANE ( 'NONE',  #3883 ) ;
#1764=AXIS2_PLACEMENT_3D ( 'NONE', #3085, #4101, #3994 ) ;
#1768=CARTESIAN_POINT ( 'NONE',  ( 19.74999999999998934, -0.001000000000001000089, -3.000000000000067946 ) ) ;
#1770=EDGE_LOOP ( 'NONE', ( #121, #7110, #7664, #5985 ) ) ;
#1780=CARTESIAN_POINT ( 'NONE',  ( -2.999999999999996447, 25.00000000000000000, 19.75000000000000000 ) ) ;
#1783=EDGE_LOOP ( 'NONE', ( #5615, #9402, #2481, #1034, #6737 ) ) ;
#1785=CYLINDRICAL_SURFACE ( 'NONE', #4035, 25.00000000000000000 ) ;
#1789=CARTESIAN_POINT ( 'NONE',  ( 1.507608415688466075E-15, 2.643749999044084920, -24.62111388750000174 ) ) ;
#1790=CARTESIAN_POINT ( 'NONE',  ( 17.67766952966369232, 1.125000000000000222, -17.67766952966369232 ) ) ;
#1793=LINE ( 'NONE', #2599, #4744 ) ;
#1797=CARTESIAN_POINT ( 'NONE',  ( -19.75000000000003197, 28.00000000000000000, -2.999999999999789946 ) ) ;
#1801=VECTOR ( 'NONE', #7530, 1000.000000000000114 ) ;
#1803=EDGE_CURVE ( 'NONE', #1671, #7292, #4784, .T. ) ;
#1809=AXIS2_PLACEMENT_3D ( 'NONE', #6300, #1014, #8778 ) ;
#1810=DIRECTION ( 'NONE',  ( -0.000000000000000000, 1.000000000000000000, -0.000000000000000000 ) ) ;
#1811=DIRECTION ( 'NONE',  ( 0.000000000000000000, 0.000000000000000000, 1.000000000000000000 ) ) ;
#1812=DIRECTION ( 'NONE',  ( 0.5000000000000012212, -0.000000000000000000, 0.8660254037844380415 ) ) ;
#1815=CIRCLE ( 'NONE', #7988, 2.999999999999997335 ) ;
#1816=VERTEX_POINT ( 'NONE', #8919 ) ;
#1824=CARTESIAN_POINT ( 'NONE',  ( 19.75000000000001066, -0.001000000000001000089, 2.999999999999927613 ) ) ;
#1828=CARTESIAN_POINT ( 'NONE',  ( 1.530808498934191521E-15, 4.862499998088169129, -25.00000000000000000 ) ) ;
#1829=DIRECTION ( 'NONE',  ( -0.5000000000000012212, 0.000000000000000000, -0.8660254037844380415 ) ) ;
#1830=VECTOR ( 'NONE', #4405, 1000.000000000000114 ) ;
#1831=VECTOR ( 'NONE', #1810, 1000.000000000000000 ) ;
#1834=CARTESIAN_POINT ( 'NONE',  ( 24.62111388750000174, 5.218749999044084653, 0.000000000000000000 ) ) ;
#1837=CARTESIAN_POINT ( 'NONE',  ( -15.75000000000003553, 25.00000000000000000, -2.999999999999832578 ) ) ;
#1841=DIRECTION ( 'NONE',  ( 2.168404344971010347E-16, -0.000000000000000000, 1.000000000000000000 ) ) ;
#1844=EDGE_LOOP ( 'NONE', ( #2368, #5001 ) ) ;
#1848=CARTESIAN_POINT ( 'NONE',  ( -17.67766952966369232, 4.237499998088169129, 17.67766952966368876 ) ) ;
#1849=CARTESIAN_POINT ( 'NONE',  ( -4.592425496802574367E-15, 0.7500000000000000000, 25.00000000000000000 ) ) ;
#1850=CARTESIAN_POINT ( 'NONE',  ( 7.874999999999916511, -0.001000000000001000089, -13.63990010960495702 ) ) ;
#1852=CARTESIAN_POINT ( 'NONE',  ( 1.530808498934191521E-15, 2.862499998088169573, -25.00000000000000000 ) ) ;
#1855=DIRECTION ( 'NONE',  ( 0.4999999999999887312, 0.000000000000000000, -0.8660254037844451469 ) ) ;
#1857=VERTEX_POINT ( 'NONE', #577 ) ;
#1858=VERTEX_POINT ( 'NONE', #3959 ) ;
#1859=ORIENTED_EDGE ( 'NONE', *, *, #8200, .F. ) ;
#1861=CARTESIAN_POINT ( 'NONE',  ( -4.592425496802574367E-15, 3.362499998088169129, 25.00000000000000000 ) ) ;
#1862=FACE_OUTER_BOUND ( 'NONE', #4884, .T. ) ;
#1864=DIRECTION ( 'NONE',  ( -0.000000000000000000, 1.000000000000000000, -0.000000000000000000 ) ) ;
#1873=ORIENTED_EDGE ( 'NONE', *, *, #1623, .T. ) ;
#1875=CARTESIAN_POINT ( 'NONE',  ( 0.000000000000000000, 85.00000000000000000, 0.000000000000000000 ) ) ;
#1878=CARTESIAN_POINT ( 'NONE',  ( 9.875000000000023093, 28.00000000000000000, 17.10400172474264835 ) ) ;
#1881=CARTESIAN_POINT ( 'NONE',  ( 17.10400172474261637, 28.00000000000000000, -9.875000000000085265 ) ) ;
#1885=CARTESIAN_POINT ( 'NONE',  ( -4.592425496802574367E-15, 1.750000000000000000, 25.00000000000000000 ) ) ;
#1886=CARTESIAN_POINT ( 'NONE',  ( -24.62111388750000884, 4.781249999044083765, 10.19839929293505421 ) ) ;
#1887=CARTESIAN_POINT ( 'NONE',  ( -24.62111388750000174, 1.893749999044084475, -3.015216831376932151E-15 ) ) ;
#1888=ORIENTED_EDGE ( 'NONE', *, *, #459, .F. ) ;
#1889=DIRECTION ( 'NONE',  ( 0.8660254037844380415, 0.000000000000000000, -0.5000000000000012212 ) ) ;
#1901=DIRECTION ( 'NONE',  ( 0.000000000000000000, 1.000000000000000000, 0.000000000000000000 ) ) ;
#1902=CARTESIAN_POINT ( 'NONE',  ( 25.00000000000000000, 3.674999998088170017, -10.35533905932737753 ) ) ;
#1903=CARTESIAN_POINT ( 'NONE',  ( -17.40975659021753330, 3.843749999044085097, 17.40975659021752975 ) ) ;
#1904=CARTESIAN_POINT ( 'NONE',  ( 0.000000000000000000, 0.000000000000000000, 0.000000000000000000 ) ) ;
#1906=CYLINDRICAL_SURFACE ( 'NONE', #8650, 2.999999999999997780 ) ;
#1912=ORIENTED_EDGE ( 'NONE', *, *, #9089, .F. ) ;
#1913=ORIENTED_EDGE ( 'NONE', *, *, #1752, .T. ) ;
#1916=AXIS2_PLACEMENT_3D ( 'NONE', #6310, #548, #4560 ) ;
#1919=CYLINDRICAL_SURFACE ( 'NONE', #7133, 2.999999999999999112 ) ;
#1920=FACE_OUTER_BOUND ( 'NONE', #7536, .T. ) ;
#1923=CARTESIAN_POINT ( 'NONE',  ( -4.592425496802574367E-15, 1.750000000000000000, 25.00000000000000000 ) ) ;
#1924=CARTESIAN_POINT ( 'NONE',  ( -24.62111388750000174, 3.831249999044084920, -10.19839929293506131 ) ) ;
#1926=AXIS2_PLACEMENT_3D ( 'NONE', #10233, #71, #10174 ) ;
#1931=CARTESIAN_POINT ( 'NONE',  ( 12.47307621135333200, -0.001000000000001000089, 15.60400172474264835 ) ) ;
#1936=CARTESIAN_POINT ( 'NONE',  ( -15.60400172474251868, 28.00000000000000000, 12.47307621135349720 ) ) ;
#1937=CARTESIAN_POINT ( 'NONE',  ( 10.19839929293506486, 4.031249999044083765, 24.62111388749999819 ) ) ;
#1942=CARTESIAN_POINT ( 'NONE',  ( 17.67766952966369232, 2.125000000000000000, -17.67766952966369232 ) ) ;
#1943=CARTESIAN_POINT ( 'NONE',  ( 10.19839929293506486, 4.031249999044083765, 24.62111388749999819 ) ) ;
#1947=CARTESIAN_POINT ( 'NONE',  ( -25.00000000000000000, 1.049999998088169129, -10.35533905932738108 ) ) ;
#1950=CYLINDRICAL_SURFACE ( 'NONE', #5363, 2.999999999999997335 ) ;
#1952=EDGE_CURVE ( 'NONE', #3209, #4627, #372, .T. ) ;
#1955=AXIS2_PLACEMENT_3D ( 'NONE', #7089, #3764, #2202 ) ;
#1960=EDGE_CURVE ( 'NONE', #3974, #5443, #9639, .T. ) ;
#1963=CARTESIAN_POINT ( 'NONE',  ( 25.00000000000000000, 2.612499998088169129, 0.000000000000000000 ) ) ;
#1964=CARTESIAN_POINT ( 'NONE',  ( 25.00000000000000000, 0.06249999999999997224, -10.35533905932737753 ) ) ;
#1965=CARTESIAN_POINT ( 'NONE',  ( -17.67766952966368876, 2.987499998088169129, -17.67766952966369232 ) ) ;
#1966=AXIS2_PLACEMENT_3D ( 'NONE', #6342, #8091, #5453 ) ;
#1968=ADVANCED_FACE ( 'NONE', ( #10409 ), #2065, .F. ) ;
#1970=CARTESIAN_POINT ( 'NONE',  ( 7.276923788646575630, -0.001000000000001000089, -18.60400172474270519 ) ) ;
#1979=EDGE_CURVE ( 'NONE', #5812, #9541, #10066, .T. ) ;
#1980=FACE_OUTER_BOUND ( 'NONE', #2514, .T. ) ;
#1983=DIRECTION ( 'NONE',  ( 0.000000000000000000, 0.000000000000000000, 1.000000000000000000 ) ) ;
#1985=CARTESIAN_POINT ( 'NONE',  ( 1.507608415688466075E-15, 3.643749999044084920, -24.62111388750000174 ) ) ;
#1986=CIRCLE ( 'NONE', #4802, 25.00000000000000000 ) ;
#1991=DIRECTION ( 'NONE',  ( -0.000000000000000000, 1.000000000000000000, 0.000000000000000000 ) ) ;
#1994=FACE_OUTER_BOUND ( 'NONE', #2153, .T. ) ;
#1995=FACE_OUTER_BOUND ( 'NONE', #7039, .T. ) ;
#1996=LINE ( 'NONE', #2087, #229 ) ;
#1997=AXIS2_PLACEMENT_3D ( 'NONE', #1600, #4986, #2576 ) ;
#1999=VECTOR ( 'NONE', #4701, 1000.000000000000000 ) ;
#2001=AXIS2_PLACEMENT_3D ( 'NONE', #8652, #7888, #5191 ) ;
#2003=CARTESIAN_POINT ( 'NONE',  ( 25.00000000000000000, 2.000000000000000000, 0.000000000000000000 ) ) ;
#2011=CARTESIAN_POINT ( 'NONE',  ( 25.00000000000000000, 0.3062499990440845643, 0.000000000000000000 ) ) ;
#2012=EDGE_CURVE ( 'NONE', #4087, #5829, #3345, .T. ) ;
#2015=EDGE_LOOP ( 'NONE', ( #809, #5825, #3140, #9910 ) ) ;
#2020=CARTESIAN_POINT ( 'NONE',  ( 17.40975659021752620, 4.268749999044085364, 17.40975659021753330 ) ) ;
#2021=CARTESIAN_POINT ( 'NONE',  ( 25.00000000000000000, 2.674999998088169129, -10.35533905932737753 ) ) ;
#2023=CARTESIAN_POINT ( 'NONE',  ( -25.00000000000000000, 1.500000000000000000, -3.061616997868383043E-15 ) ) ;
#2024=FACE_BOUND ( 'NONE', #9135, .T. ) ;
#2027=DIRECTION ( 'NONE',  ( 0.000000000000000000, 1.000000000000000000, -0.000000000000000000 ) ) ;
#2030=CARTESIAN_POINT ( 'NONE',  ( -12.47307621135311351, -0.001000000000001000089, 15.60400172474282599 ) ) ;
#2031=ORIENTED_EDGE ( 'NONE', *, *, #9706, .T. ) ;
#2032=VERTEX_POINT ( 'NONE', #8639 ) ;
#2033=EDGE_CURVE ( 'NONE', #8288, #8662, #4463, .T. ) ;
#2037=CARTESIAN_POINT ( 'NONE',  ( 10.19839929293506486, 5.206249999044084475, 24.62111388749999819 ) ) ;
#2039=ADVANCED_FACE ( 'NONE', ( #1028 ), #252, .F. ) ;
#2042=DIRECTION ( 'NONE',  ( 0.000000000000000000, 1.000000000000000000, 0.000000000000000000 ) ) ;
#2043=CARTESIAN_POINT ( 'NONE',  ( 0.000000000000000000, 85.00000000000000000, 0.000000000000000000 ) ) ;
#2047=ORIENTED_EDGE ( 'NONE', *, *, #8553, .T. ) ;
#2048=CARTESIAN_POINT ( 'NONE',  ( 12.13990010960493748, 25.00000000000000000, 10.47307621135328759 ) ) ;
#2049=DIRECTION ( 'NONE',  ( -0.4999999999999888978, 0.000000000000000000, 0.8660254037844450359 ) ) ;
#2055=DIRECTION ( 'NONE',  ( -0.000000000000000000, 1.000000000000000000, -0.000000000000000000 ) ) ;
#2056=ORIENTED_EDGE ( 'NONE', *, *, #4452, .F. ) ;
#2058=CARTESIAN_POINT ( 'NONE',  ( -17.40975659021753330, 3.018749999044084475, 17.40975659021752975 ) ) ;
#2060=CARTESIAN_POINT ( 'NONE',  ( -25.00000000000001421, 3.562500000000000444, 10.35533905932737397 ) ) ;
#2061=( LENGTH_UNIT ( ) NAMED_UNIT ( * ) SI_UNIT ( .MILLI., .METRE. ) );
#2064=CARTESIAN_POINT ( 'NONE',  ( 0.000000000000000000, 27.99999999999999645, 0.000000000000000000 ) ) ;
#2065=PLANE ( 'NONE',  #8127 ) ;
#2066=EDGE_CURVE ( 'NONE', #2242, #93, #4883, .T. ) ;
#2067=VERTEX_POINT ( 'NONE', #7156 ) ;
#2069=VERTEX_POINT ( 'NONE', #2271 ) ;
#2070=VERTEX_POINT ( 'NONE', #3138 ) ;
#2071=EDGE_CURVE ( 'NONE', #93, #8568, #614, .T. ) ;
#2072=FACE_OUTER_BOUND ( 'NONE', #9479, .T. ) ;
#2073=CARTESIAN_POINT ( 'NONE',  ( -3.957930336368489021E-15, -0.001000000000001000089, -19.75000000000000000 ) ) ;
#2077=CARTESIAN_POINT ( 'NONE',  ( 19.75000000000000000, 25.00000000000000000, -7.291468677852036884E-14 ) ) ;
#2082=LINE ( 'NONE', #10695, #2667 ) ;
#2087=CARTESIAN_POINT ( 'NONE',  ( 15.60400172474260927, 28.00000000000000000, -12.47307621135339062 ) ) ;
#2088=CARTESIAN_POINT ( 'NONE',  ( 12.13990010960486288, 28.00000000000000000, -10.47307621135337641 ) ) ;
#2091=ORIENTED_EDGE ( 'NONE', *, *, #5927, .F. ) ;
#2094=CARTESIAN_POINT ( 'NONE',  ( 24.62111388749999108, 1.331249999044084475, 10.19839929293507730 ) ) ;
#2095=ORIENTED_EDGE ( 'NONE', *, *, #8426, .F. ) ;
#2101=ORIENTED_EDGE ( 'NONE', *, *, #10844, .T. ) ;
#2102=VERTEX_POINT ( 'NONE', #9890 ) ;
#2103=EDGE_LOOP ( 'NONE', ( #8861, #8120, #5100, #2746 ) ) ;
#2106=CARTESIAN_POINT ( 'NONE',  ( 24.62111388750000174, 1.456249999044084475, -10.19839929293505776 ) ) ;
#2107=CARTESIAN_POINT ( 'NONE',  ( 10.35533905932738286, 4.812500000000000888, 24.99999999999999645 ) ) ;
#2109=DIRECTION ( 'NONE',  ( -0.000000000000000000, 1.000000000000000000, -0.000000000000000000 ) ) ;
#2111=LINE ( 'NONE', #8959, #551 ) ;
#2112=DIRECTION ( 'NONE',  ( -0.8660254037844380415, -0.000000000000000000, 0.5000000000000012212 ) ) ;
#2117=EDGE_LOOP ( 'NONE', ( #111, #6362 ) ) ;
#2121=CARTESIAN_POINT ( 'NONE',  ( 12.47307621135322186, 25.00000000000000000, -15.60400172474273717 ) ) ;
#2122=ORIENTED_EDGE ( 'NONE', *, *, #9952, .F. ) ;
#2127=AXIS2_PLACEMENT_3D ( 'NONE', #7839, #4481, #1811 ) ;
#2133=DIRECTION ( 'NONE',  ( -0.000000000000000000, -1.000000000000000000, -0.000000000000000000 ) ) ;
#2140=VECTOR ( 'NONE', #6811, 1000.000000000000114 ) ;
#2145=CARTESIAN_POINT ( 'NONE',  ( 24.62111388749999108, 3.331249999044084920, 10.19839929293507730 ) ) ;
#2146=ORIENTED_EDGE ( 'NONE', *, *, #6976, .F. ) ;
#2153=EDGE_LOOP ( 'NONE', ( #9436, #3932, #7844, #3822 ) ) ;
#2155=ORIENTED_EDGE ( 'NONE', *, *, #2390, .F. ) ;
#2160=VECTOR ( 'NONE', #7045, 1000.000000000000000 ) ;
#2161=CARTESIAN_POINT ( 'NONE',  ( 24.62111388750000174, 2.456249999044084475, -10.19839929293505776 ) ) ;
#2162=CARTESIAN_POINT ( 'NONE',  ( 24.99999999999999289, 2.937500000000000444, 10.35533905932739529 ) ) ;
#2163=PRESENTATION_STYLE_ASSIGNMENT (( #8956 ) ) ;
#2164=( BOUNDED_CURVE ( )  B_SPLINE_CURVE ( 2, ( #9323, #5151, #8500, #5215, #8558, #1005, #5423, #284, #10497 ),
 .UNSPECIFIED., .F., .F. ) 
 B_SPLINE_CURVE_WITH_KNOTS ( ( 3, 2, 2, 2, 3 ),
 ( 0.5500000000000000444, 0.5749999999999999556, 0.5999999999999999778, 0.6250000000000000000, 0.6500000000000000222 ),
 .UNSPECIFIED. ) 
 CURVE ( )  GEOMETRIC_REPRESENTATION_ITEM ( )  RATIONAL_B_SPLINE_CURVE ( ( 1.000000000000000000, 0.9238795325112867385, 1.000000000000000000, 0.9238795325112867385, 1.000000000000000000, 0.9238795325112867385, 1.000000000000000000, 0.9238795325112867385, 1.000000000000000000 ) ) 
 REPRESENTATION_ITEM ( '' )  );
#2165=DIRECTION ( 'NONE',  ( 0.000000000000000000, 1.000000000000000000, 0.000000000000000000 ) ) ;
#2166=CARTESIAN_POINT ( 'NONE',  ( 25.00000000000000000, 1.612499998088169351, 0.000000000000000000 ) ) ;
#2169=CARTESIAN_POINT ( 'NONE',  ( 1.530808498934191521E-15, 1.250000000000000000, -25.00000000000000000 ) ) ;
#2171=AXIS2_PLACEMENT_3D ( 'NONE', #10827, #10710, #7441 ) ;
#2175=VECTOR ( 'NONE', #5832, 1000.000000000000000 ) ;
#2176=DIRECTION ( 'NONE',  ( -0.8660254037844433705, 0.000000000000000000, -0.4999999999999916733 ) ) ;
#2177=AXIS2_PLACEMENT_3D ( 'NONE', #56, #9267, #1709 ) ;
#2181=CARTESIAN_POINT ( 'NONE',  ( -7.875000000000116351, 28.00000000000000000, -13.63990010960484334 ) ) ;
#2182=ORIENTED_EDGE ( 'NONE', *, *, #4781, .T. ) ;
#2187=AXIS2_PLACEMENT_3D ( 'NONE', #7889, #1040, #3735 ) ;
#2191=ADVANCED_FACE ( 'NONE', ( #3038 ), #4775, .F. ) ;
#2193=CARTESIAN_POINT ( 'NONE',  ( -4.592425496802574367E-15, 4.362499998088169129, 25.00000000000000000 ) ) ;
#2196=EDGE_CURVE ( 'NONE', #6472, #7410, #6285, .T. ) ;
#2199=CARTESIAN_POINT ( 'NONE',  ( -24.62111388750000884, 3.956249999044084475, 10.19839929293505421 ) ) ;
#2200=VERTEX_POINT ( 'NONE', #7249 ) ;
#2202=DIRECTION ( 'NONE',  ( 0.000000000000000000, 0.000000000000000000, 1.000000000000000000 ) ) ;
#2209=ADVANCED_FACE ( 'NONE', ( #2429 ), #5811, .F. ) ;
#2213=CARTESIAN_POINT ( 'NONE',  ( -10.19839929293507552, 3.081249999044084475, 24.62111388749999463 ) ) ;
#2214=CARTESIAN_POINT ( 'NONE',  ( -10.35533905932737575, 4.312500000000000888, -25.00000000000000000 ) ) ;
#2216=CARTESIAN_POINT ( 'NONE',  ( -25.00000000000001421, 1.174999998088169351, 10.35533905932737397 ) ) ;
#2218=DIRECTION ( 'NONE',  ( -0.000000000000000000, -1.000000000000000000, -0.000000000000000000 ) ) ;
#2221=ORIENTED_EDGE ( 'NONE', *, *, #7234, .T. ) ;
#2229=CARTESIAN_POINT ( 'NONE',  ( -15.13990010960484867, -0.001000000000001000089, 5.276923788646865177 ) ) ;
#2231=CARTESIAN_POINT ( 'NONE',  ( 9.875000000000023093, 25.00000000000000000, 20.10400172474264835 ) ) ;
#2235=CARTESIAN_POINT ( 'NONE',  ( -15.60400172474278158, -0.001000000000001000089, -12.47307621135316680 ) ) ;
#2236=CARTESIAN_POINT ( 'NONE',  ( 17.67766952966369232, 4.737499998088169129, -17.67766952966369232 ) ) ;
#2239=VECTOR ( 'NONE', #86, 1000.000000000000000 ) ;
#2240=ORIENTED_EDGE ( 'NONE', *, *, #3251, .T. ) ;
#2242=VERTEX_POINT ( 'NONE', #2583 ) ;
#2244=MECHANICAL_DESIGN_GEOMETRIC_PRESENTATION_REPRESENTATION('',(#1029),#6496);
#2246=CARTESIAN_POINT ( 'NONE',  ( -4.522825247065398226E-15, 5.143749999044084475, 24.62111388750000174 ) ) ;
#2247=ORIENTED_EDGE ( 'NONE', *, *, #4315, .T. ) ;
#2252=VERTEX_POINT ( 'NONE', #6758 ) ;
#2254=DIRECTION ( 'NONE',  ( 0.000000000000000000, 1.000000000000000000, -0.000000000000000000 ) ) ;
#2255=CARTESIAN_POINT ( 'NONE',  ( 17.40975659021752975, 3.343749999044085097, -17.40975659021752975 ) ) ;
#2257=ORIENTED_EDGE ( 'NONE', *, *, #4852, .T. ) ;
#2263=DIRECTION ( 'NONE',  ( -0.4999999999999947820, 0.000000000000000000, 0.8660254037844417052 ) ) ;
#2264=CARTESIAN_POINT ( 'NONE',  ( 24.62111388750000174, 2.218749999044084653, 0.000000000000000000 ) ) ;
#2265=ORIENTED_EDGE ( 'NONE', *, *, #7955, .T. ) ;
#2271=CARTESIAN_POINT ( 'NONE',  ( 24.62111388750000174, 0.2187499990440845699, 0.000000000000000000 ) ) ;
#2272=DIRECTION ( 'NONE',  ( -0.000000000000000000, -1.000000000000000000, -0.000000000000000000 ) ) ;
#2274=EDGE_CURVE ( 'NONE', #5054, #5784, #9331, .T. ) ;
#2276=ORIENTED_EDGE ( 'NONE', *, *, #8540, .T. ) ;
#2277=ORIENTED_EDGE ( 'NONE', *, *, #4796, .F. ) ;
#2286=DIRECTION ( 'NONE',  ( -0.4999999999999947820, 0.000000000000000000, 0.8660254037844417052 ) ) ;
#2289=VERTEX_POINT ( 'NONE', #4207 ) ;
#2292=VERTEX_POINT ( 'NONE', #8349 ) ;
#2293=FACE_OUTER_BOUND ( 'NONE', #8366, .T. ) ;
#2294=DIRECTION ( 'NONE',  ( -0.000000000000000000, 1.000000000000000000, -0.000000000000000000 ) ) ;
#2295=LINE ( 'NONE', #3105, #6783 ) ;
#2298=CARTESIAN_POINT ( 'NONE',  ( 25.00000000000000000, -2.710505431213761085E-17, 0.000000000000000000 ) ) ;
#2300=ORIENTED_EDGE ( 'NONE', *, *, #3755, .T. ) ;
#2301=ORIENTED_EDGE ( 'NONE', *, *, #2735, .T. ) ;
#2305=CARTESIAN_POINT ( 'NONE',  ( 24.62111388749999108, 2.331249999044084475, 10.19839929293507730 ) ) ;
#2309=CARTESIAN_POINT ( 'NONE',  ( -9.874999999999777955, 25.00000000000000000, 17.10400172474279401 ) ) ;
#2311=ORIENTED_EDGE ( 'NONE', *, *, #4227, .F. ) ;
#2312=ORIENTED_EDGE ( 'NONE', *, *, #1390, .T. ) ;
#2317=CARTESIAN_POINT ( 'NONE',  ( -17.40975659021752975, 1.593749999044084431, -17.40975659021752975 ) ) ;
#2321=EDGE_CURVE ( 'NONE', #5377, #9220, #9117, .T. ) ;
#2322=DIRECTION ( 'NONE',  ( -1.000000000000000000, 0.000000000000000000, 3.708321773340234242E-15 ) ) ;
#2323=CARTESIAN_POINT ( 'NONE',  ( 5.276923788646705304, -0.001000000000001000089, 15.13990010960490196 ) ) ;
#2326=CIRCLE ( 'NONE', #932, 10.50000000000000000 ) ;
#2327=VERTEX_POINT ( 'NONE', #7570 ) ;
#2328=ORIENTED_EDGE ( 'NONE', *, *, #2747, .F. ) ;
#2331=AXIS2_PLACEMENT_3D ( 'NONE', #4299, #6011, #7718 ) ;
#2334=CARTESIAN_POINT ( 'NONE',  ( 10.19839929293506486, 1.031249999044084653, 24.62111388749999819 ) ) ;
#2336=EDGE_CURVE ( 'NONE', #7939, #3078, #10843, .T. ) ;
#2342=VERTEX_POINT ( 'NONE', #10170 ) ;
#2344=ORIENTED_EDGE ( 'NONE', *, *, #8352, .F. ) ;
#2345=VECTOR ( 'NONE', #7624, 1000.000000000000000 ) ;
#2346=VECTOR ( 'NONE', #7492, 1000.000000000000114 ) ;
#2350=CARTESIAN_POINT ( 'NONE',  ( -18.60400172474257730, -0.001000000000001000089, 7.276923788646904256 ) ) ;
#2351=AXIS2_PLACEMENT_3D ( 'NONE', #8822, #2042, #6348 ) ;
#2352=CARTESIAN_POINT ( 'NONE',  ( -12.13990010960478827, -0.001000000000001000089, 10.47307621135345990 ) ) ;
#2353=DIRECTION ( 'NONE',  ( 0.4999999999999917288, 0.000000000000000000, -0.8660254037844434816 ) ) ;
#2354=FACE_OUTER_BOUND ( 'NONE', #2117, .T. ) ;
#2357=EDGE_CURVE ( 'NONE', #2862, #5242, #7519, .T. ) ;
#2361=CARTESIAN_POINT ( 'NONE',  ( -10.19839929293505776, 4.706249999044084475, -24.62111388750000174 ) ) ;
#2367=CARTESIAN_POINT ( 'NONE',  ( 24.62111388750000174, 2.281249999044085541, -10.19839929293505776 ) ) ;
#2368=ORIENTED_EDGE ( 'NONE', *, *, #9748, .T. ) ;
#2373=CARTESIAN_POINT ( 'NONE',  ( -24.62111388750000174, 0.6562499990440846531, -10.19839929293506131 ) ) ;
#2374=ORIENTED_EDGE ( 'NONE', *, *, #2357, .T. ) ;
#2375=DIRECTION ( 'NONE',  ( 0.000000000000000000, 0.000000000000000000, 1.000000000000000000 ) ) ;
#2376=CARTESIAN_POINT ( 'NONE',  ( 12.13990010960486288, -0.001000000000001000089, -10.47307621135337641 ) ) ;
#2378=CARTESIAN_POINT ( 'NONE',  ( 0.000000000000000000, 31.00000000000000000, 0.000000000000000000 ) ) ;
#2381=ORIENTED_EDGE ( 'NONE', *, *, #3014, .T. ) ;
#2385=CARTESIAN_POINT ( 'NONE',  ( -4.522825247065398226E-15, 3.143749999044084475, 24.62111388750000174 ) ) ;
#2386=CARTESIAN_POINT ( 'NONE',  ( -24.62111388750000884, 1.781249999044084431, 10.19839929293505421 ) ) ;
#2390=EDGE_CURVE ( 'NONE', #8735, #9894, #669, .T. ) ;
#2393=LINE ( 'NONE', #8302, #2866 ) ;
#2412=AXIS2_PLACEMENT_3D ( 'NONE', #8935, #2955, #2049 ) ;
#2413=DIRECTION ( 'NONE',  ( 0.000000000000000000, 0.000000000000000000, 1.000000000000000000 ) ) ;
#2414=CARTESIAN_POINT ( 'NONE',  ( -10.19839929293507375, 1.906249999044084431, 24.62111388749999108 ) ) ;
#2419=LINE ( 'NONE', #4098, #8658 ) ;
#2421=CARTESIAN_POINT ( 'NONE',  ( 10.19839929293505953, 0.4062499990440845421, -24.62111388750000174 ) ) ;
#2422=LINE ( 'NONE', #7563, #3179 ) ;
#2426=LINE ( 'NONE', #2376, #7361 ) ;
#2429=FACE_OUTER_BOUND ( 'NONE', #5241, .T. ) ;
#2432=ORIENTED_EDGE ( 'NONE', *, *, #2864, .F. ) ;
#2434=CARTESIAN_POINT ( 'NONE',  ( 24.62111388749999463, 2.331249999044084031, 10.19839929293507730 ) ) ;
#2438=CARTESIAN_POINT ( 'NONE',  ( 3.061616997868383043E-15, 85.00000000000000000, 25.00000000000000000 ) ) ;
#2443=ORIENTED_EDGE ( 'NONE', *, *, #9275, .F. ) ;
#2444=EDGE_LOOP ( 'NONE', ( #7564, #8051, #4091, #10854, #7436 ) ) ;
#2447=DIRECTION ( 'NONE',  ( -0.000000000000000000, -1.000000000000000000, -0.000000000000000000 ) ) ;
#2453=AXIS2_PLACEMENT_3D ( 'NONE', #6251, #6192, #10329 ) ;
#2455=EDGE_CURVE ( 'NONE', #3294, #10189, #6532, .T. ) ;
#2457=VECTOR ( 'NONE', #9370, 1000.000000000000000 ) ;
#2464=DIRECTION ( 'NONE',  ( 0.000000000000000000, 1.000000000000000000, 0.000000000000000000 ) ) ;
#2466=CARTESIAN_POINT ( 'NONE',  ( 10.19839929293505953, 0.4062499990440845421, -24.62111388750000174 ) ) ;
#2468=VERTEX_POINT ( 'NONE', #683 ) ;
#2469=EDGE_CURVE ( 'NONE', #10189, #9894, #6826, .T. ) ;
#2471=CARTESIAN_POINT ( 'NONE',  ( 18.60400172474263414, 25.00000000000000000, -7.276923788646775471 ) ) ;
#2472=CARTESIAN_POINT ( 'NONE',  ( -4.522825247065398226E-15, 2.968749999044084653, 24.62111388750000174 ) ) ;
#2473=PLANE ( 'NONE',  #389 ) ;
#2480=AXIS2_PLACEMENT_3D ( 'NONE', #4339, #7703, #134 ) ;
#2481=ORIENTED_EDGE ( 'NONE', *, *, #9857, .F. ) ;
#2482=AXIS2_PLACEMENT_3D ( 'NONE', #10057, #10897, #9225 ) ;
#2483=CARTESIAN_POINT ( 'NONE',  ( -24.62111388750000174, 2.831249999044084475, -10.19839929293506131 ) ) ;
#2484=CARTESIAN_POINT ( 'NONE',  ( -24.62111388750000174, 1.656249999044084431, -10.19839929293506131 ) ) ;
#2489=DIRECTION ( 'NONE',  ( -0.000000000000000000, -1.000000000000000000, -0.000000000000000000 ) ) ;
#2492=ORIENTED_EDGE ( 'NONE', *, *, #5927, .T. ) ;
#2493=ORIENTED_EDGE ( 'NONE', *, *, #6940, .F. ) ;
#2500=DIRECTION ( 'NONE',  ( -0.5000000000000073275, 0.000000000000000000, -0.8660254037844343777 ) ) ;
#2502=( BOUNDED_CURVE ( )  B_SPLINE_CURVE ( 2, ( #1828, #3344, #5210, #8552, #6740, #10101, #1703, #329, #4497 ),
 .UNSPECIFIED., .F., .F. ) 
 B_SPLINE_CURVE_WITH_KNOTS ( ( 3, 2, 2, 2, 3 ),
 ( 0.8500000000000000888, 0.8750000000000001110, 0.9000000000000001332, 0.9250000000000001554, 0.9500000000000000666 ),
 .UNSPECIFIED. ) 
 CURVE ( )  GEOMETRIC_REPRESENTATION_ITEM ( )  RATIONAL_B_SPLINE_CURVE ( ( 0.9999999999999996669, 0.9238795325112870716, 1.000000000000000000, 0.9238795325112867385, 1.000000000000000000, 0.9238795325112867385, 1.000000000000000000, 0.9238795325112864054, 1.000000000000000444 ) ) 
 REPRESENTATION_ITEM ( '' )  );
#2505=AXIS2_PLACEMENT_3D ( 'NONE', #4584, #2889, #6288 ) ;
#2508=ORIENTED_EDGE ( 'NONE', *, *, #469, .F. ) ;
#2511=DIRECTION ( 'NONE',  ( 0.000000000000000000, 0.000000000000000000, 1.000000000000000000 ) ) ;
#2512=DIRECTION ( 'NONE',  ( -0.000000000000000000, -1.000000000000000000, -0.000000000000000000 ) ) ;
#2514=EDGE_LOOP ( 'NONE', ( #5798, #10625, #2240, #2915 ) ) ;
#2515=CARTESIAN_POINT ( 'NONE',  ( -2.999999999999999112, -0.001000000000001000089, -19.75000000000000000 ) ) ;
#2516=DIRECTION ( 'NONE',  ( 0.000000000000000000, 1.000000000000000000, 0.000000000000000000 ) ) ;
#2517=ORIENTED_EDGE ( 'NONE', *, *, #5576, .F. ) ;
#2520=CARTESIAN_POINT ( 'NONE',  ( 24.62111388750000174, 5.218749999044084653, 0.000000000000000000 ) ) ;
#2522=ORIENTED_EDGE ( 'NONE', *, *, #3539, .T. ) ;
#2526=CARTESIAN_POINT ( 'NONE',  ( 17.40975659021752975, 4.343749999044084653, -17.40975659021752975 ) ) ;
#2529=DIRECTION ( 'NONE',  ( 0.000000000000000000, 0.000000000000000000, 1.000000000000000000 ) ) ;
#2531=CARTESIAN_POINT ( 'NONE',  ( 18.60400172474268032, 25.00000000000000000, 7.276923788646642244 ) ) ;
#2532=DIRECTION ( 'NONE',  ( 0.000000000000000000, 1.000000000000000000, 0.000000000000000000 ) ) ;
#2533=CYLINDRICAL_SURFACE ( 'NONE', #2482, 10.50000000000000000 ) ;
#2536=EDGE_LOOP ( 'NONE', ( #9626, #7411, #6470, #3601 ) ) ;
#2538=CARTESIAN_POINT ( 'NONE',  ( -18.60400172474273361, -0.001000000000001000089, -7.276923788646511682 ) ) ;
#2540=CARTESIAN_POINT ( 'NONE',  ( 10.19839929293505953, 1.581249999044084475, -24.62111388750000174 ) ) ;
#2541=CARTESIAN_POINT ( 'NONE',  ( -17.67766952966369232, 0.6250000000000000000, 17.67766952966368876 ) ) ;
#2547=CARTESIAN_POINT ( 'NONE',  ( -3.000000000000000888, 28.00000000000000000, -15.75000000000000355 ) ) ;
#2561=CARTESIAN_POINT ( 'NONE',  ( 0.000000000000000000, 8.000000000000003553, 0.000000000000000000 ) ) ;
#2562=DIRECTION ( 'NONE',  ( 0.000000000000000000, 0.000000000000000000, -1.000000000000000000 ) ) ;
#2565=ORIENTED_EDGE ( 'NONE', *, *, #9839, .F. ) ;
#2566=DIRECTION ( 'NONE',  ( 0.000000000000000000, 0.000000000000000000, 1.000000000000000000 ) ) ;
#2570=LINE ( 'NONE', #1768, #10387 ) ;
#2576=DIRECTION ( 'NONE',  ( 0.000000000000000000, 0.000000000000000000, 1.000000000000000000 ) ) ;
#2578=DIRECTION ( 'NONE',  ( -0.000000000000000000, -1.000000000000000000, -0.000000000000000000 ) ) ;
#2579=CARTESIAN_POINT ( 'NONE',  ( -5.276923788646491253, -0.001000000000001000089, 15.13990010960497834 ) ) ;
#2583=CARTESIAN_POINT ( 'NONE',  ( -4.592425496802574367E-15, 3.750000000000000000, 25.00000000000000000 ) ) ;
#2590=ORIENTED_EDGE ( 'NONE', *, *, #261, .F. ) ;
#2591=AXIS2_PLACEMENT_3D ( 'NONE', #5397, #3033, #7925 ) ;
#2593=DIRECTION ( 'NONE',  ( -2.168404344971010347E-16, 0.000000000000000000, -1.000000000000000000 ) ) ;
#2596=CARTESIAN_POINT ( 'NONE',  ( 17.40975659021752975, 1.518749999044084698, -17.40975659021752975 ) ) ;
#2597=CARTESIAN_POINT ( 'NONE',  ( -4.522825247065398226E-15, 2.968749999044084653, 24.62111388750000174 ) ) ;
#2598=LINE ( 'NONE', #5338, #848 ) ;
#2599=CARTESIAN_POINT ( 'NONE',  ( -3.223142256880076948E-15, -0.001000000000001000089, -12.75000000000000178 ) ) ;
#2600=CARTESIAN_POINT ( 'NONE',  ( 7.276923788646707969, 25.00000000000000000, 18.60400172474265190 ) ) ;
#2601=VECTOR ( 'NONE', #7327, 1000.000000000000000 ) ;
#2604=CARTESIAN_POINT ( 'NONE',  ( -9.874999999999777955, 25.00000000000000000, 17.10400172474279401 ) ) ;
#2607=ORIENTED_EDGE ( 'NONE', *, *, #10639, .F. ) ;
#2608=LINE ( 'NONE', #5349, #5434 ) ;
#2609=ADVANCED_FACE ( 'NONE', ( #2715, #6166 ), #7051, .F. ) ;
#2613=DIRECTION ( 'NONE',  ( -0.000000000000000000, -1.000000000000000000, -0.000000000000000000 ) ) ;
#2615=LINE ( 'NONE', #4352, #7412 ) ;
#2619=CARTESIAN_POINT ( 'NONE',  ( -19.75000000000003197, -0.001000000000001000089, -2.999999999999789946 ) ) ;
#2621=CYLINDRICAL_SURFACE ( 'NONE', #8239, 25.00000000000000000 ) ;
#2622=CARTESIAN_POINT ( 'NONE',  ( -3.223142256880076948E-15, 25.00000000000000000, -15.75000000000000000 ) ) ;
#2624=CIRCLE ( 'NONE', #6213, 25.00000000000000000 ) ;
#2625=AXIS2_PLACEMENT_3D ( 'NONE', #7300, #8958, #7247 ) ;
#2626=DIRECTION ( 'NONE',  ( 0.8660254037844362651, 0.000000000000000000, -0.5000000000000041078 ) ) ;
#2627=CARTESIAN_POINT ( 'NONE',  ( -24.62111388750000174, 4.718749999044084653, -3.015216831376932151E-15 ) ) ;
#2640=PLANE ( 'NONE',  #572 ) ;
#2647=CARTESIAN_POINT ( 'NONE',  ( -10.19839929293505776, 0.7062499990440844755, -24.62111388750000174 ) ) ;
#2648=AXIS2_PLACEMENT_3D ( 'NONE', #6097, #2578, #4377 ) ;
#2650=EDGE_CURVE ( 'NONE', #2786, #9703, #10750, .T. ) ;
#2651=CARTESIAN_POINT ( 'NONE',  ( -4.592425496802574367E-15, 4.362499998088169129, 25.00000000000000000 ) ) ;
#2652=CARTESIAN_POINT ( 'NONE',  ( 17.40975659021752620, 5.093749999044084653, 17.40975659021753330 ) ) ;
#2653=CARTESIAN_POINT ( 'NONE',  ( -4.592425496802574367E-15, 3.362499998088169129, 25.00000000000000000 ) ) ;
#2655=DIRECTION ( 'NONE',  ( 2.168404344971010347E-16, -0.000000000000000000, 1.000000000000000000 ) ) ;
#2656=FACE_BOUND ( 'NONE', #8999, .T. ) ;
#2662=ORIENTED_EDGE ( 'NONE', *, *, #646, .F. ) ;
#2665=CARTESIAN_POINT ( 'NONE',  ( 10.47307621135324496, -0.001000000000001000089, -12.13990010960497479 ) ) ;
#2667=VECTOR ( 'NONE', #4745, 1000.000000000000000 ) ;
#2676=ADVANCED_FACE ( 'NONE', ( #3609 ), #1906, .F. ) ;
#2677=EDGE_LOOP ( 'NONE', ( #10778, #9981, #6427, #3056 ) ) ;
#2679=AXIS2_PLACEMENT_3D ( 'NONE', #2891, #8537, #7837 ) ;
#2680=ORIENTED_EDGE ( 'NONE', *, *, #3251, .F. ) ;
#2681=AXIS2_PLACEMENT_3D ( 'NONE', #6108, #1901, #6877 ) ;
#2684=CARTESIAN_POINT ( 'NONE',  ( 3.000000000000000888, 28.00000000000000000, 15.75000000000000355 ) ) ;
#2686=VERTEX_POINT ( 'NONE', #6997 ) ;
#2691=ADVANCED_FACE ( 'NONE', ( #6053, #2882, #9352, #8637, #4461, #2656, #8525, #974, #7702, #10354, #133, #9414, #3494, #6882 ), #192, .F. ) ;
#2693=CARTESIAN_POINT ( 'NONE',  ( 7.276923788646707969, 25.00000000000000000, 18.60400172474265190 ) ) ;
#2694=CIRCLE ( 'NONE', #10821, 2.999999999999999112 ) ;
#2698=CARTESIAN_POINT ( 'NONE',  ( 1.507608415688466075E-15, 4.468749999044084653, -24.62111388750000174 ) ) ;
#2701=CARTESIAN_POINT ( 'NONE',  ( -10.35533905932737575, 0.9249999980881692396, -25.00000000000000000 ) ) ;
#2702=CARTESIAN_POINT ( 'NONE',  ( 10.35533905932738641, 1.799999998088168685, -24.99999999999999289 ) ) ;
#2703=FACE_BOUND ( 'NONE', #3986, .T. ) ;
#2706=DIRECTION ( 'NONE',  ( 0.000000000000000000, 0.000000000000000000, 1.000000000000000000 ) ) ;
#2710=LINE ( 'NONE', #2538, #9138 ) ;
#2713=CARTESIAN_POINT ( 'NONE',  ( -4.592425496802574367E-15, 2.362499998088169129, 25.00000000000000000 ) ) ;
#2714=CARTESIAN_POINT ( 'NONE',  ( 10.19839929293505953, 3.406249999044085097, -24.62111388750000174 ) ) ;
#2715=FACE_BOUND ( 'NONE', #400, .T. ) ;
#2717=DIRECTION ( 'NONE',  ( -0.000000000000000000, -1.000000000000000000, -0.000000000000000000 ) ) ;
#2721=EDGE_LOOP ( 'NONE', ( #9336, #6495, #7057, #3540 ) ) ;
#2727=LINE ( 'NONE', #6834, #7121 ) ;
#2733=CARTESIAN_POINT ( 'NONE',  ( -17.67766952966368876, 1.375000000000000000, -17.67766952966369232 ) ) ;
#2735=EDGE_CURVE ( 'NONE', #6733, #2289, #7394, .T. ) ;
#2739=FACE_OUTER_BOUND ( 'NONE', #9020, .T. ) ;
#2741=DIRECTION ( 'NONE',  ( 0.000000000000000000, 0.000000000000000000, -1.000000000000000000 ) ) ;
#2745=CARTESIAN_POINT ( 'NONE',  ( 17.40975659021752620, 4.093749999044084653, 17.40975659021753330 ) ) ;
#2746=ORIENTED_EDGE ( 'NONE', *, *, #1960, .F. ) ;
#2747=EDGE_CURVE ( 'NONE', #5785, #5770, #527, .T. ) ;
#2750=CARTESIAN_POINT ( 'NONE',  ( 24.62111388750000174, 4.218749999044084653, 0.000000000000000000 ) ) ;
#2751=CARTESIAN_POINT ( 'NONE',  ( -24.62111388750000174, 0.8937499990440845865, -3.015216831376932151E-15 ) ) ;
#2752=ORIENTED_EDGE ( 'NONE', *, *, #936, .F. ) ;
#2753=CARTESIAN_POINT ( 'NONE',  ( -15.60400172474251868, -0.001000000000001000089, 12.47307621135349720 ) ) ;
#2756=DIRECTION ( 'NONE',  ( 0.000000000000000000, 0.000000000000000000, 1.000000000000000000 ) ) ;
#2763=CARTESIAN_POINT ( 'NONE',  ( -17.67766952966368876, 4.987499998088170017, -17.67766952966369232 ) ) ;
#2764=CARTESIAN_POINT ( 'NONE',  ( 1.507608415688466075E-15, 4.468749999044084653, -24.62111388750000174 ) ) ;
#2766=DIRECTION ( 'NONE',  ( 0.000000000000000000, 1.000000000000000000, 0.000000000000000000 ) ) ;
#2774=DIRECTION ( 'NONE',  ( 0.5000000000000042188, 0.000000000000000000, 0.8660254037844362651 ) ) ;
#2776=VECTOR ( 'NONE', #1829, 999.9999999999998863 ) ;
#2780=LINE ( 'NONE', #6176, #258 ) ;
#2782=CYLINDRICAL_SURFACE ( 'NONE', #5536, 10.50000000000000000 ) ;
#2784=CARTESIAN_POINT ( 'NONE',  ( 3.061616997868383043E-15, 85.00000000000000000, 25.00000000000000000 ) ) ;
#2785=CARTESIAN_POINT ( 'NONE',  ( 1.507608415688466075E-15, 4.643749999044084475, -24.62111388750000174 ) ) ;
#2786=VERTEX_POINT ( 'NONE', #10518 ) ;
#2788=CIRCLE ( 'NONE', #3301, 25.00000000000000000 ) ;
#2797=DIRECTION ( 'NONE',  ( -0.000000000000000000, 1.000000000000000000, 0.000000000000000000 ) ) ;
#2798=DIRECTION ( 'NONE',  ( 0.000000000000000000, 0.000000000000000000, 1.000000000000000000 ) ) ;
#2799=ADVANCED_FACE ( 'NONE', ( #5652 ), #8659, .F. ) ;
#2800=ORIENTED_EDGE ( 'NONE', *, *, #7971, .T. ) ;
#2805=CARTESIAN_POINT ( 'NONE',  ( 5.276923788646596947, -0.001000000000001000089, -15.13990010960494459 ) ) ;
#2806=VERTEX_POINT ( 'NONE', #7842 ) ;
#2807=EDGE_CURVE ( 'NONE', #10131, #4266, #10239, .T. ) ;
#2815=VECTOR ( 'NONE', #10825, 1000.000000000000000 ) ;
#2816=EDGE_LOOP ( 'NONE', ( #1467, #3149 ) ) ;
#2822=CARTESIAN_POINT ( 'NONE',  ( 17.67766952966368521, 3.487499998088169129, 17.67766952966369232 ) ) ;
#2824=AXIS2_PLACEMENT_3D ( 'NONE', #2561, #5956, #9312 ) ;
#2832=VECTOR ( 'NONE', #7350, 1000.000000000000000 ) ;
#2835=DIRECTION ( 'NONE',  ( 0.8660254037844433705, 0.000000000000000000, 0.4999999999999916733 ) ) ;
#2836=FACE_OUTER_BOUND ( 'NONE', #2536, .T. ) ;
#2841=CARTESIAN_POINT ( 'NONE',  ( -10.35533905932737220, 1.687500000000000222, 25.00000000000001421 ) ) ;
#2842=CARTESIAN_POINT ( 'NONE',  ( -24.62111388750000884, 4.956249999044084475, 10.19839929293505421 ) ) ;
#2843=AXIS2_PLACEMENT_3D ( 'NONE', #1682, #9961, #803 ) ;
#2846=SURFACE_STYLE_FILL_AREA ( #4545 ) ;
#2850=DIRECTION ( 'NONE',  ( -0.000000000000000000, -1.000000000000000000, -0.000000000000000000 ) ) ;
#2852=AXIS2_PLACEMENT_3D ( 'NONE', #7620, #9391, #4320 ) ;
#2854=AXIS2_PLACEMENT_3D ( 'NONE', #4009, #3960, #3902 ) ;
#2858=VECTOR ( 'NONE', #10634, 1000.000000000000000 ) ;
#2860=CARTESIAN_POINT ( 'NONE',  ( -17.67766952966368876, 0.3750000000000000000, -17.67766952966369232 ) ) ;
#2862=VERTEX_POINT ( 'NONE', #6525 ) ;
#2864=EDGE_CURVE ( 'NONE', #10373, #10312, #9709, .T. ) ;
#2866=VECTOR ( 'NONE', #9292, 1000.000000000000000 ) ;
#2868=CARTESIAN_POINT ( 'NONE',  ( 17.67766952966368521, 2.487499998088169129, 17.67766952966369232 ) ) ;
#2871=CIRCLE ( 'NONE', #8166, 2.999999999999997780 ) ;
#2874=VECTOR ( 'NONE', #9459, 1000.000000000000000 ) ;
#2875=CARTESIAN_POINT ( 'NONE',  ( 1.530808498934191521E-15, 0.2500000000000000000, -25.00000000000000000 ) ) ;
#2877=CARTESIAN_POINT ( 'NONE',  ( 1.507608415688466075E-15, 4.643749999044085364, -24.62111388750000174 ) ) ;
#2879=CARTESIAN_POINT ( 'NONE',  ( -4.592425496802574367E-15, 2.750000000000000000, 25.00000000000000000 ) ) ;
#2881=FACE_OUTER_BOUND ( 'NONE', #8570, .T. ) ;
#2882=FACE_BOUND ( 'NONE', #10230, .T. ) ;
#2889=DIRECTION ( 'NONE',  ( -0.000000000000000000, 1.000000000000000000, 0.000000000000000000 ) ) ;
#2891=CARTESIAN_POINT ( 'NONE',  ( -9.874999999999777955, -0.001000000000001000089, 17.10400172474279401 ) ) ;
#2893=CARTESIAN_POINT ( 'NONE',  ( -17.10400172474275848, -0.001000000000001000089, -9.874999999999836575 ) ) ;
#2900=DIRECTION ( 'NONE',  ( -0.8660254037844361541, 0.000000000000000000, 0.5000000000000042188 ) ) ;
#2914=EDGE_CURVE ( 'NONE', #10312, #7767, #6475, .T. ) ;
#2915=ORIENTED_EDGE ( 'NONE', *, *, #3317, .F. ) ;
#2916=ORIENTED_EDGE ( 'NONE', *, *, #1066, .T. ) ;
#2920=CARTESIAN_POINT ( 'NONE',  ( 17.40975659021752975, 3.518749999044084920, -17.40975659021752975 ) ) ;
#2921=CARTESIAN_POINT ( 'NONE',  ( -25.00000000000000000, 4.500000000000000888, -3.061616997868383043E-15 ) ) ;
#2927=CARTESIAN_POINT ( 'NONE',  ( 17.67766952966369232, 0.7374999980881691286, -17.67766952966369232 ) ) ;
#2931=VERTEX_POINT ( 'NONE', #4150 ) ;
#2932=EDGE_CURVE ( 'NONE', #5856, #1858, #6581, .T. ) ;
#2937=ADVANCED_FACE ( 'NONE', ( #9829 ), #10776, .F. ) ;
#2938=FACE_OUTER_BOUND ( 'NONE', #4343, .T. ) ;
#2941=FACE_OUTER_BOUND ( 'NONE', #10377, .T. ) ;
#2943=EDGE_CURVE ( 'NONE', #1427, #10373, #2419, .T. ) ;
#2946=AXIS2_PLACEMENT_3D ( 'NONE', #3941, #509, #7198 ) ;
#2950=CARTESIAN_POINT ( 'NONE',  ( 25.00000000000000000, 5.000000000000000000, 0.000000000000000000 ) ) ;
#2954=DIRECTION ( 'NONE',  ( 0.000000000000000000, 1.000000000000000000, 0.000000000000000000 ) ) ;
#2955=DIRECTION ( 'NONE',  ( 0.000000000000000000, 1.000000000000000000, 0.000000000000000000 ) ) ;
#2956=CARTESIAN_POINT ( 'NONE',  ( -24.62111388750000174, 4.831249999044084475, -10.19839929293506131 ) ) ;
#2960=CARTESIAN_POINT ( 'NONE',  ( 15.60400172474269453, -0.001000000000001000089, 12.47307621135327693 ) ) ;
#2968=CARTESIAN_POINT ( 'NONE',  ( 17.67766952966369232, 1.737499998088169351, -17.67766952966369232 ) ) ;
#2971=CARTESIAN_POINT ( 'NONE',  ( 24.62111388750000174, 3.393749999044084475, 0.000000000000000000 ) ) ;
#2972=VERTEX_POINT ( 'NONE', #8952 ) ;
#2973=CARTESIAN_POINT ( 'NONE',  ( 24.99999999999999289, 1.937500000000000000, 10.35533905932739529 ) ) ;
#2975=CARTESIAN_POINT ( 'NONE',  ( -25.00000000000000000, 1.049999998088169129, -10.35533905932738108 ) ) ;
#2976=FACE_OUTER_BOUND ( 'NONE', #7574, .T. ) ;
#2977=CARTESIAN_POINT ( 'NONE',  ( 25.00000000000000000, 1.000000000000000000, 0.000000000000000000 ) ) ;
#2979=AXIS2_PLACEMENT_3D ( 'NONE', #10058, #4993, #3242 ) ;
#2985=CARTESIAN_POINT ( 'NONE',  ( -15.75000000000000000, 28.00000000000000000, 1.681956355172181189E-13 ) ) ;
#2986=CIRCLE ( 'NONE', #8460, 2.999999999999997335 ) ;
#2989=CARTESIAN_POINT ( 'NONE',  ( 0.000000000000000000, 20.00000000000000355, 20.00000000000000000 ) ) ;
#2992=FACE_OUTER_BOUND ( 'NONE', #8759, .T. ) ;
#2994=CARTESIAN_POINT ( 'NONE',  ( 0.000000000000000000, 85.00000000000000000, 0.000000000000000000 ) ) ;
#3005=AXIS2_PLACEMENT_3D ( 'NONE', #7212, #10580, #2286 ) ;
#3011=CARTESIAN_POINT ( 'NONE',  ( -19.74999999999996803, 25.00000000000000000, 3.000000000000206057 ) ) ;
#3012=CARTESIAN_POINT ( 'NONE',  ( 1.530808498934191521E-15, 0.2500000000000000000, -25.00000000000000000 ) ) ;
#3013=CARTESIAN_POINT ( 'NONE',  ( 19.75000000000001066, -0.001000000000001000089, 2.999999999999927613 ) ) ;
#3014=EDGE_CURVE ( 'NONE', #849, #2806, #10214, .T. ) ;
#3015=EDGE_LOOP ( 'NONE', ( #10006, #2344, #5681, #10885 ) ) ;
#3023=ORIENTED_EDGE ( 'NONE', *, *, #9075, .F. ) ;
#3027=VECTOR ( 'NONE', #10579, 1000.000000000000000 ) ;
#3031=CARTESIAN_POINT ( 'NONE',  ( 1.507608415688466075E-15, 2.643749999044084920, -24.62111388750000174 ) ) ;
#3032=CARTESIAN_POINT ( 'NONE',  ( -17.67766952966368876, 2.375000000000000000, -17.67766952966369232 ) ) ;
#3033=DIRECTION ( 'NONE',  ( 1.000000000000000000, 0.000000000000000000, -2.168404344971010347E-16 ) ) ;
#3034=VECTOR ( 'NONE', #8788, 1000.000000000000114 ) ;
#3036=CARTESIAN_POINT ( 'NONE',  ( -12.47307621135344391, 28.00000000000000000, -15.60400172474256131 ) ) ;
#3037=VECTOR ( 'NONE', #3855, 1000.000000000000000 ) ;
#3038=FACE_OUTER_BOUND ( 'NONE', #9876, .T. ) ;
#3040=ORIENTED_EDGE ( 'NONE', *, *, #5386, .F. ) ;
#3043=CARTESIAN_POINT ( 'NONE',  ( -25.00000000000001066, 4.562500000000001776, 10.35533905932737397 ) ) ;
#3044=DIRECTION ( 'NONE',  ( -0.000000000000000000, 1.000000000000000000, 0.000000000000000000 ) ) ;
#3055=EDGE_CURVE ( 'NONE', #6443, #3821, #9868, .T. ) ;
#3056=ORIENTED_EDGE ( 'NONE', *, *, #921, .F. ) ;
#3059=CARTESIAN_POINT ( 'NONE',  ( 25.00000000000000000, 4.612499998088169129, 0.000000000000000000 ) ) ;
#3060=EDGE_CURVE ( 'NONE', #3974, #3699, #7736, .T. ) ;
#3063=FACE_OUTER_BOUND ( 'NONE', #2015, .T. ) ;
#3068=DIRECTION ( 'NONE',  ( 0.000000000000000000, 1.000000000000000000, 0.000000000000000000 ) ) ;
#3069=CARTESIAN_POINT ( 'NONE',  ( -4.522825247065398226E-15, 4.143749999044083587, 24.62111388750000174 ) ) ;
#3076=EDGE_CURVE ( 'NONE', #2342, #1227, #6858, .T. ) ;
#3078=VERTEX_POINT ( 'NONE', #6030 ) ;
#3082=CARTESIAN_POINT ( 'NONE',  ( 15.60400172474269453, 28.00000000000000000, 12.47307621135327693 ) ) ;
#3083=CARTESIAN_POINT ( 'NONE',  ( -24.62111388750000174, 1.718749999044084431, -3.015216831376932151E-15 ) ) ;
#3085=CARTESIAN_POINT ( 'NONE',  ( -19.74999999999996803, -0.001000000000001000089, 3.000000000000206057 ) ) ;
#3086=DIRECTION ( 'NONE',  ( -0.5000000000000073275, 0.000000000000000000, -0.8660254037844343777 ) ) ;
#3089=CARTESIAN_POINT ( 'NONE',  ( -4.592425496802574367E-15, 3.362499998088169129, 25.00000000000000000 ) ) ;
#3091=ORIENTED_EDGE ( 'NONE', *, *, #3837, .T. ) ;
#3092=ORIENTED_EDGE ( 'NONE', *, *, #5873, .F. ) ;
#3095=( NAMED_UNIT ( * ) SI_UNIT ( $, .STERADIAN. ) SOLID_ANGLE_UNIT ( ) );
#3100=VERTEX_POINT ( 'NONE', #5089 ) ;
#3101=EDGE_LOOP ( 'NONE', ( #3790, #360, #8467, #8814 ) ) ;
#3104=CARTESIAN_POINT ( 'NONE',  ( -10.47307621135341904, 25.00000000000000000, -12.13990010960482557 ) ) ;
#3105=CARTESIAN_POINT ( 'NONE',  ( 24.62111388750000174, 5.306249999044084120, 0.000000000000000000 ) ) ;
#3106=CARTESIAN_POINT ( 'NONE',  ( 1.530808498934191521E-15, 0.2500000000000000000, -25.00000000000000000 ) ) ;
#3110=EDGE_LOOP ( 'NONE', ( #3092, #10508, #4136, #10819 ) ) ;
#3112=CARTESIAN_POINT ( 'NONE',  ( 0.000000000000000000, 8.000000000000000000, 0.000000000000000000 ) ) ;
#3115=CARTESIAN_POINT ( 'NONE',  ( 10.19839929293505953, 4.581249999044083587, -24.62111388750000174 ) ) ;
#3125=VERTEX_POINT ( 'NONE', #5214 ) ;
#3128=VECTOR ( 'NONE', #8401, 1000.000000000000000 ) ;
#3132=CARTESIAN_POINT ( 'NONE',  ( -24.62111388750000174, 3.656249999044084653, -10.19839929293506131 ) ) ;
#3133=ORIENTED_EDGE ( 'NONE', *, *, #2336, .F. ) ;
#3138=CARTESIAN_POINT ( 'NONE',  ( 24.62111388750000174, 0.3937499990440845310, 0.000000000000000000 ) ) ;
#3140=ORIENTED_EDGE ( 'NONE', *, *, #7546, .T. ) ;
#3144=UNCERTAINTY_MEASURE_WITH_UNIT (LENGTH_MEASURE( 1.000000000000000082E-05 ), #2061, 'distance_accuracy_value', 'NONE');
#3145=CARTESIAN_POINT ( 'NONE',  ( 10.19839929293505953, 2.406249999044085541, -24.62111388750000174 ) ) ;
#3148=EDGE_CURVE ( 'NONE', #9311, #416, #7119, .T. ) ;
#3149=ORIENTED_EDGE ( 'NONE', *, *, #1144, .F. ) ;
#3150=LINE ( 'NONE', #7257, #3027 ) ;
#3154=VECTOR ( 'NONE', #6023, 1000.000000000000000 ) ;
#3158=CYLINDRICAL_SURFACE ( 'NONE', #8497, 25.00000000000000000 ) ;
#3159=CARTESIAN_POINT ( 'NONE',  ( 1.285879139104720831E-15, 28.00000000000000000, 10.50000000000000000 ) ) ;
#3160=FACE_OUTER_BOUND ( 'NONE', #1685, .T. ) ;
#3161=CIRCLE ( 'NONE', #3891, 2.999999999999997335 ) ;
#3163=FACE_BOUND ( 'NONE', #8399, .T. ) ;
#3164=DIRECTION ( 'NONE',  ( 4.710179996720586888E-17, 0.9230769230769232392, -0.3846153846153844702 ) ) ;
#3165=ORIENTED_EDGE ( 'NONE', *, *, #6990, .T. ) ;
#3166=ORIENTED_EDGE ( 'NONE', *, *, #4102, .T. ) ;
#3169=AXIS2_PLACEMENT_3D ( 'NONE', #8755, #9353, #6883 ) ;
#3170=CARTESIAN_POINT ( 'NONE',  ( -10.19839929293507375, 4.081249999044084475, 24.62111388749999108 ) ) ;
#3171=LINE ( 'NONE', #6568, #2815 ) ;
#3179=VECTOR ( 'NONE', #890, 1000.000000000000114 ) ;
#3183=CARTESIAN_POINT ( 'NONE',  ( 24.62111388749999463, 5.331249999044085364, 10.19839929293507730 ) ) ;
#3188=CARTESIAN_POINT ( 'NONE',  ( 0.000000000000000000, 85.00000000000000000, 0.000000000000000000 ) ) ;
#3193=ORIENTED_EDGE ( 'NONE', *, *, #3399, .F. ) ;
#3196=EDGE_LOOP ( 'NONE', ( #678, #8307, #2680, #1613 ) ) ;
#3200=AXIS2_PLACEMENT_3D ( 'NONE', #7516, #8563, #1011 ) ;
#3202=CARTESIAN_POINT ( 'NONE',  ( -18.60400172474257730, -0.001000000000001000089, 7.276923788646904256 ) ) ;
#3209=VERTEX_POINT ( 'NONE', #7909 ) ;
#3218=CARTESIAN_POINT ( 'NONE',  ( 2.999999999999997335, 25.00000000000000000, -15.75000000000000355 ) ) ;
#3219=LINE ( 'NONE', #644, #9579 ) ;
#3225=VERTEX_POINT ( 'NONE', #2048 ) ;
#3227=DIRECTION ( 'NONE',  ( -0.000000000000000000, -1.000000000000000000, -0.000000000000000000 ) ) ;
#3228=DIRECTION ( 'NONE',  ( -2.168404344971010594E-16, 0.000000000000000000, -1.000000000000000000 ) ) ;
#3234=CARTESIAN_POINT ( 'NONE',  ( 24.62111388750000174, 2.281249999044085541, -10.19839929293505776 ) ) ;
#3235=DIRECTION ( 'NONE',  ( 0.000000000000000000, 0.000000000000000000, 1.000000000000000000 ) ) ;
#3242=DIRECTION ( 'NONE',  ( 0.4999999999999887312, 0.000000000000000000, -0.8660254037844451469 ) ) ;
#3244=ORIENTED_EDGE ( 'NONE', *, *, #8832, .T. ) ;
#3246=ORIENTED_EDGE ( 'NONE', *, *, #7494, .F. ) ;
#3249=CARTESIAN_POINT ( 'NONE',  ( -17.40975659021753330, 1.018749999044084698, 17.40975659021752975 ) ) ;
#3250=CARTESIAN_POINT ( 'NONE',  ( -24.62111388750000884, 0.7812499990440845421, 10.19839929293505421 ) ) ;
#3251=EDGE_CURVE ( 'NONE', #7713, #4798, #4069, .T. ) ;
#3253=VERTEX_POINT ( 'NONE', #5320 ) ;
#3255=FACE_OUTER_BOUND ( 'NONE', #4356, .T. ) ;
#3258=CARTESIAN_POINT ( 'NONE',  ( -3.223142256880076948E-15, 28.00000000000000000, -12.75000000000000178 ) ) ;
#3259=ADVANCED_FACE ( 'NONE', ( #1119 ), #7084, .F. ) ;
#3260=ORIENTED_EDGE ( 'NONE', *, *, #10223, .F. ) ;
#3263=APPLICATION_CONTEXT ( 'automotive_design' ) ;
#3270=CARTESIAN_POINT ( 'NONE',  ( 10.35533905932738286, 3.812500000000000000, 24.99999999999999645 ) ) ;
#3273=EDGE_LOOP ( 'NONE', ( #4492, #8232, #635, #233 ) ) ;
#3274=CARTESIAN_POINT ( 'NONE',  ( 17.67766952966368521, 4.875000000000000000, 17.67766952966369232 ) ) ;
#3278=ORIENTED_EDGE ( 'NONE', *, *, #5211, .T. ) ;
#3279=DIRECTION ( 'NONE',  ( 0.000000000000000000, 1.000000000000000000, -0.000000000000000000 ) ) ;
#3285=CARTESIAN_POINT ( 'NONE',  ( -17.40975659021752975, 2.593749999044084653, -17.40975659021752975 ) ) ;
#3292=CARTESIAN_POINT ( 'NONE',  ( -10.19839929293507552, 2.906249999044085541, 24.62111388749999463 ) ) ;
#3294=VERTEX_POINT ( 'NONE', #3590 ) ;
#3300=DIRECTION ( 'NONE',  ( -2.168404344971010347E-16, 0.000000000000000000, -1.000000000000000000 ) ) ;
#3301=AXIS2_PLACEMENT_3D ( 'NONE', #3188, #5752, #7568 ) ;
#3303=VERTEX_POINT ( 'NONE', #6979 ) ;
#3305=CARTESIAN_POINT ( 'NONE',  ( 10.19839929293505953, 0.5812499990440844755, -24.62111388750000174 ) ) ;
#3314=CARTESIAN_POINT ( 'NONE',  ( -17.67766952966369232, 3.625000000000000000, 17.67766952966368876 ) ) ;
#3317=EDGE_CURVE ( 'NONE', #1227, #4798, #6142, .T. ) ;
#3319=ORIENTED_EDGE ( 'NONE', *, *, #10452, .T. ) ;
#3321=ORIENTED_EDGE ( 'NONE', *, *, #6800, .F. ) ;
#3327=LINE ( 'NONE', #5076, #7126 ) ;
#3331=EDGE_CURVE ( 'NONE', #9311, #1064, #8988, .T. ) ;
#3333=EDGE_CURVE ( 'NONE', #8063, #10373, #3861, .T. ) ;
#3336=CARTESIAN_POINT ( 'NONE',  ( -25.00000000000001066, 4.174999998088169129, 10.35533905932737397 ) ) ;
#3344=CARTESIAN_POINT ( 'NONE',  ( -10.35533905932741128, 4.924999998088170905, -24.99999999999996803 ) ) ;
#3345=CIRCLE ( 'NONE', #5, 2.999999999999997335 ) ;
#3351=CARTESIAN_POINT ( 'NONE',  ( 10.19839929293505953, 4.406249999044084653, -24.62111388750000174 ) ) ;
#3352=CYLINDRICAL_SURFACE ( 'NONE', #2852, 28.00000000000000000 ) ;
#3354=DIRECTION ( 'NONE',  ( -0.5000000000000012212, 0.000000000000000000, -0.8660254037844380415 ) ) ;
#3356=CARTESIAN_POINT ( 'NONE',  ( -7.875000000000116351, 25.00000000000000000, -10.63990010960484334 ) ) ;
#3357=FACE_OUTER_BOUND ( 'NONE', #6154, .T. ) ;
#3362=EDGE_LOOP ( 'NONE', ( #8190, #2276, #9559, #580 ) ) ;
#3363=ORIENTED_EDGE ( 'NONE', *, *, #10874, .T. ) ;
#3364=VERTEX_POINT ( 'NONE', #489 ) ;
#3366=CYLINDRICAL_SURFACE ( 'NONE', #7208, 25.00000000000000000 ) ;
#3368=AXIS2_PLACEMENT_3D ( 'NONE', #7177, #4383, #4599 ) ;
#3369=CARTESIAN_POINT ( 'NONE',  ( -12.47307621135311351, 28.00000000000000000, 15.60400172474282599 ) ) ;
#3370=CARTESIAN_POINT ( 'NONE',  ( -19.74999999999996803, -0.001000000000001000089, 3.000000000000206057 ) ) ;
#3372=DIRECTION ( 'NONE',  ( 0.5000000000000012212, 0.000000000000000000, 0.8660254037844380415 ) ) ;
#3373=DIRECTION ( 'NONE',  ( 0.000000000000000000, 0.000000000000000000, 1.000000000000000000 ) ) ;
#3375=AXIS2_PLACEMENT_3D ( 'NONE', #10383, #2797, #4801 ) ;
#3377=VECTOR ( 'NONE', #1812, 999.9999999999998863 ) ;
#3378=VERTEX_POINT ( 'NONE', #10658 ) ;
#3380=AXIS2_PLACEMENT_3D ( 'NONE', #1313, #2133, #4697 ) ;
#3381=LINE ( 'NONE', #2665, #486 ) ;
#3382=CIRCLE ( 'NONE', #1457, 2.999999999999998668 ) ;
#3383=AXIS2_PLACEMENT_3D ( 'NONE', #7422, #10018, #10803 ) ;
#3387=CYLINDRICAL_SURFACE ( 'NONE', #6238, 2.999999999999997335 ) ;
#3388=FACE_OUTER_BOUND ( 'NONE', #9334, .T. ) ;
#3392=EDGE_CURVE ( 'NONE', #3734, #5443, #3977, .T. ) ;
#3393=CIRCLE ( 'NONE', #953, 2.999999999999997335 ) ;
#3394=ORIENTED_EDGE ( 'NONE', *, *, #5056, .F. ) ;
#3397=CARTESIAN_POINT ( 'NONE',  ( 7.875000000000019540, -0.001000000000001000089, 13.63990010960489840 ) ) ;
#3398=CARTESIAN_POINT ( 'NONE',  ( 1.530808498934191521E-15, 3.862499998088169573, -25.00000000000000000 ) ) ;
#3399=EDGE_CURVE ( 'NONE', #6044, #241, #5330, .T. ) ;
#3400=DIRECTION ( 'NONE',  ( -0.000000000000000000, 1.000000000000000000, -0.000000000000000000 ) ) ;
#3403=LINE ( 'NONE', #941, #7781 ) ;
#3407=LINE ( 'NONE', #2693, #2776 ) ;
#3409=ORIENTED_EDGE ( 'NONE', *, *, #4385, .T. ) ;
#3417=FACE_OUTER_BOUND ( 'NONE', #4288, .T. ) ;
#3420=CARTESIAN_POINT ( 'NONE',  ( 13.63990010960487353, -0.001000000000001000089, -7.875000000000067502 ) ) ;
#3426=CARTESIAN_POINT ( 'NONE',  ( 2.999999999999999112, -0.001000000000001000089, 19.75000000000000000 ) ) ;
#3429=CARTESIAN_POINT ( 'NONE',  ( 25.00000000000000000, 5.612499998088169129, 0.000000000000000000 ) ) ;
#3430=CARTESIAN_POINT ( 'NONE',  ( -4.522825247065398226E-15, 3.968749999044084209, 24.62111388750000174 ) ) ;
#3431=DIRECTION ( 'NONE',  ( 0.000000000000000000, 0.000000000000000000, 1.000000000000000000 ) ) ;
#3432=ORIENTED_EDGE ( 'NONE', *, *, #5735, .F. ) ;
#3443=CARTESIAN_POINT ( 'NONE',  ( -17.10400172474275848, 28.00000000000000000, -9.874999999999836575 ) ) ;
#3446=CARTESIAN_POINT ( 'NONE',  ( 10.47307621135333200, 28.00000000000000000, 12.13990010960489840 ) ) ;
#3451=PRODUCT_DEFINITION ( 'UNKNOWN', '', #6353, #7052 ) ;
#3453=DIRECTION ( 'NONE',  ( 1.000000000000000000, 0.000000000000000000, 0.000000000000000000 ) ) ;
#3455=CARTESIAN_POINT ( 'NONE',  ( 25.00000000000000000, 5.612499998088169129, 0.000000000000000000 ) ) ;
#3456=CARTESIAN_POINT ( 'NONE',  ( 18.60400172474268032, 25.00000000000000000, 7.276923788646641356 ) ) ;
#3458=DIRECTION ( 'NONE',  ( -0.8660254037844434816, 0.000000000000000000, -0.4999999999999918399 ) ) ;
#3467=DIRECTION ( 'NONE',  ( -1.000000000000000000, 0.000000000000000000, 3.708321773340234242E-15 ) ) ;
#3468=CARTESIAN_POINT ( 'NONE',  ( 24.62111388750000174, 4.281249999044084653, -10.19839929293505776 ) ) ;
#3471=CARTESIAN_POINT ( 'NONE',  ( -19.74999999999996803, 28.00000000000000000, 3.000000000000206057 ) ) ;
#3472=ADVANCED_FACE ( 'NONE', ( #36 ), #8320, .F. ) ;
#3480=ORIENTED_EDGE ( 'NONE', *, *, #508, .F. ) ;
#3482=ORIENTED_EDGE ( 'NONE', *, *, #10855, .T. ) ;
#3484=CIRCLE ( 'NONE', #3851, 2.999999999999996891 ) ;
#3485=DIRECTION ( 'NONE',  ( 0.000000000000000000, 1.000000000000000000, 0.000000000000000000 ) ) ;
#3488=CARTESIAN_POINT ( 'NONE',  ( -24.62111388750000174, 2.893749999044084475, -3.015216831376932151E-15 ) ) ;
#3489=CARTESIAN_POINT ( 'NONE',  ( -10.19839929293505776, 3.531249999044084653, -24.62111388750000174 ) ) ;
#3490=DIRECTION ( 'NONE',  ( 0.000000000000000000, 1.000000000000000000, -0.000000000000000000 ) ) ;
#3491=EDGE_CURVE ( 'NONE', #883, #8678, #7592, .T. ) ;
#3493=CARTESIAN_POINT ( 'NONE',  ( 2.999999999999996447, 25.00000000000000000, -19.75000000000000000 ) ) ;
#3494=FACE_OUTER_BOUND ( 'NONE', #750, .T. ) ;
#3497=VECTOR ( 'NONE', #5808, 1000.000000000000000 ) ;
#3501=VERTEX_POINT ( 'NONE', #4421 ) ;
#3504=PLANE ( 'NONE',  #5612 ) ;
#3509=CARTESIAN_POINT ( 'NONE',  ( -15.13990010960496235, 25.00000000000000000, -5.276923788646544544 ) ) ;
#3510=CARTESIAN_POINT ( 'NONE',  ( 0.000000000000000000, 0.000000000000000000, 0.000000000000000000 ) ) ;
#3513=EDGE_LOOP ( 'NONE', ( #900, #2101, #9843, #1391 ) ) ;
#3516=CARTESIAN_POINT ( 'NONE',  ( -17.10400172474254532, 25.00000000000000000, 9.875000000000202505 ) ) ;
#3517=CARTESIAN_POINT ( 'NONE',  ( -25.00000000000000000, 4.112499998088169129, -3.061616997868383043E-15 ) ) ;
#3526=AXIS2_PLACEMENT_3D ( 'NONE', #3629, #8720, #1163 ) ;
#3532=CARTESIAN_POINT ( 'NONE',  ( -25.00000000000000000, 1.112499998088169351, -3.061616997868383043E-15 ) ) ;
#3533=CARTESIAN_POINT ( 'NONE',  ( 10.35533905932738286, 1.424999998088169129, 24.99999999999999645 ) ) ;
#3539=EDGE_CURVE ( 'NONE', #10806, #5726, #4245, .T. ) ;
#3540=ORIENTED_EDGE ( 'NONE', *, *, #8344, .F. ) ;
#3543=FACE_OUTER_BOUND ( 'NONE', #10485, .T. ) ;
#3545=CARTESIAN_POINT ( 'NONE',  ( 17.40975659021752975, 0.5187499990440846975, -17.40975659021752975 ) ) ;
#3546=CARTESIAN_POINT ( 'NONE',  ( -25.00000000000000000, 5.112499998088170017, -3.061616997868383043E-15 ) ) ;
#3547=CARTESIAN_POINT ( 'NONE',  ( 10.19839929293506486, 4.031249999044083765, 24.62111388749999819 ) ) ;
#3548=PLANE ( 'NONE',  #7547 ) ;
#3552=EDGE_CURVE ( 'NONE', #5695, #7304, #5138, .T. ) ;
#3558=ORIENTED_EDGE ( 'NONE', *, *, #9439, .T. ) ;
#3561=EDGE_CURVE ( 'NONE', #2252, #7275, #1748, .T. ) ;
#3564=DIRECTION ( 'NONE',  ( 0.000000000000000000, 1.000000000000000000, 0.000000000000000000 ) ) ;
#3565=ORIENTED_EDGE ( 'NONE', *, *, #9583, .F. ) ;
#3569=CARTESIAN_POINT ( 'NONE',  ( 3.223142256880076948E-15, 25.00000000000000000, 15.75000000000000000 ) ) ;
#3571=CYLINDRICAL_SURFACE ( 'NONE', #10462, 25.00000000000000000 ) ;
#3572=CARTESIAN_POINT ( 'NONE',  ( -17.40975659021753330, 5.018749999044084475, 17.40975659021752975 ) ) ;
#3575=AXIS2_PLACEMENT_3D ( 'NONE', #2309, #9985, #2413 ) ;
#3576=ADVANCED_FACE ( 'NONE', ( #6441 ), #7849, .F. ) ;
#3577=VERTEX_POINT ( 'NONE', #3955 ) ;
#3581=FACE_OUTER_BOUND ( 'NONE', #7448, .T. ) ;
#3584=FACE_OUTER_BOUND ( 'NONE', #10661, .T. ) ;
#3585=LINE ( 'NONE', #1936, #5517 ) ;
#3586=FACE_OUTER_BOUND ( 'NONE', #8888, .T. ) ;
#3590=CARTESIAN_POINT ( 'NONE',  ( 5.276923788646705304, 25.00000000000000000, 15.13990010960490196 ) ) ;
#3595=FACE_OUTER_BOUND ( 'NONE', #9895, .T. ) ;
#3596=CARTESIAN_POINT ( 'NONE',  ( -25.00000000000001066, 2.562500000000000444, 10.35533905932737397 ) ) ;
#3598=DIRECTION ( 'NONE',  ( -0.8660254037844431485, 0.000000000000000000, -0.4999999999999922839 ) ) ;
#3600=ORIENTED_EDGE ( 'NONE', *, *, #4315, .F. ) ;
#3601=ORIENTED_EDGE ( 'NONE', *, *, #10945, .F. ) ;
#3602=ORIENTED_EDGE ( 'NONE', *, *, #10048, .T. ) ;
#3603=FACE_OUTER_BOUND ( 'NONE', #7170, .T. ) ;
#3605=CARTESIAN_POINT ( 'NONE',  ( -19.74999999999996803, 28.00000000000000000, 3.000000000000206057 ) ) ;
#3606=CARTESIAN_POINT ( 'NONE',  ( 1.530808498934191521E-15, 4.862499998088169129, -25.00000000000000000 ) ) ;
#3607=CARTESIAN_POINT ( 'NONE',  ( -10.19839929293507552, 2.906249999044085541, 24.62111388749999463 ) ) ;
#3609=FACE_OUTER_BOUND ( 'NONE', #538, .T. ) ;
#3612=CYLINDRICAL_SURFACE ( 'NONE', #10472, 25.00000000000000000 ) ;
#3613=EDGE_LOOP ( 'NONE', ( #6889, #1348 ) ) ;
#3615=ORIENTED_EDGE ( 'NONE', *, *, #10700, .F. ) ;
#3616=EDGE_CURVE ( 'NONE', #241, #8189, #7254, .T. ) ;
#3623=CARTESIAN_POINT ( 'NONE',  ( 0.000000000000000000, 31.00000000000000000, -10.50000000000000000 ) ) ;
#3625=CARTESIAN_POINT ( 'NONE',  ( 17.10400172474269098, 25.00000000000000000, 9.874999999999957367 ) ) ;
#3629=CARTESIAN_POINT ( 'NONE',  ( 0.000000000000000000, 0.000000000000000000, 0.000000000000000000 ) ) ;
#3631=ORIENTED_EDGE ( 'NONE', *, *, #8540, .F. ) ;
#3634=EDGE_CURVE ( 'NONE', #8678, #883, #2624, .T. ) ;
#3638=VERTEX_POINT ( 'NONE', #3369 ) ;
#3646=CARTESIAN_POINT ( 'NONE',  ( 10.35533905932737930, 2.187500000000000444, -25.00000000000000000 ) ) ;
#3648=CARTESIAN_POINT ( 'NONE',  ( -17.40975659021752975, 0.7687499990440845865, -17.40975659021752975 ) ) ;
#3652=CARTESIAN_POINT ( 'NONE',  ( -10.35533905932737575, 2.312500000000000888, -25.00000000000000000 ) ) ;
#3653=FACE_OUTER_BOUND ( 'NONE', #4025, .T. ) ;
#3654=CARTESIAN_POINT ( 'NONE',  ( 0.000000000000000000, 8.000000000000000000, 0.000000000000000000 ) ) ;
#3655=( BOUNDED_CURVE ( )  B_SPLINE_CURVE ( 2, ( #2298, #10872, #8159, #3971, #3106 ),
 .UNSPECIFIED., .F., .F. ) 
 B_SPLINE_CURVE_WITH_KNOTS ( ( 3, 2, 3 ),
 ( 0.000000000000000000, 0.02500000000000000486, 0.05000000000000000971 ),
 .UNSPECIFIED. ) 
 CURVE ( )  GEOMETRIC_REPRESENTATION_ITEM ( )  RATIONAL_B_SPLINE_CURVE ( ( 1.000000000000000000, 0.9238795325112867385, 1.000000000000000000, 0.9238795325112867385, 1.000000000000000000 ) ) 
 REPRESENTATION_ITEM ( '' )  );
#3657=EDGE_LOOP ( 'NONE', ( #8206, #6387, #3244, #10682 ) ) ;
#3659=ORIENTED_EDGE ( 'NONE', *, *, #10086, .F. ) ;
#3663=CARTESIAN_POINT ( 'NONE',  ( 1.530808498934191521E-15, 2.862499998088169573, -25.00000000000000000 ) ) ;
#3664=CARTESIAN_POINT ( 'NONE',  ( -17.67766952966368876, 0.3750000000000000000, -17.67766952966369232 ) ) ;
#3665=( LENGTH_UNIT ( ) NAMED_UNIT ( * ) SI_UNIT ( .MILLI., .METRE. ) );
#3671=DIRECTION ( 'NONE',  ( -0.000000000000000000, -1.000000000000000000, -0.000000000000000000 ) ) ;
#3679=AXIS2_PLACEMENT_3D ( 'NONE', #6756, #4205, #1550 ) ;
#3680=DIRECTION ( 'NONE',  ( -0.4999999999999917288, 0.000000000000000000, 0.8660254037844434816 ) ) ;
#3681=DIRECTION ( 'NONE',  ( -0.000000000000000000, 1.000000000000000000, -0.000000000000000000 ) ) ;
#3682=DIRECTION ( 'NONE',  ( -0.000000000000000000, -1.000000000000000000, -0.000000000000000000 ) ) ;
#3689=ADVANCED_FACE ( 'NONE', ( #9900 ), #9284, .F. ) ;
#3690=ORIENTED_EDGE ( 'NONE', *, *, #8287, .T. ) ;
#3691=SURFACE_STYLE_USAGE ( .BOTH. , #7901 ) ;
#3693=DIRECTION ( 'NONE',  ( 0.4999999999999947820, 0.000000000000000000, -0.8660254037844417052 ) ) ;
#3699=VERTEX_POINT ( 'NONE', #1294 ) ;
#3701=AXIS2_PLACEMENT_3D ( 'NONE', #5044, #3940, #4828 ) ;
#3703=CARTESIAN_POINT ( 'NONE',  ( 15.75000000000000000, 28.00000000000000000, -5.821397334365942453E-14 ) ) ;
#3705=VECTOR ( 'NONE', #9949, 1000.000000000000000 ) ;
#3708=FACE_OUTER_BOUND ( 'NONE', #9958, .T. ) ;
#3715=ORIENTED_EDGE ( 'NONE', *, *, #10471, .F. ) ;
#3716=VECTOR ( 'NONE', #2263, 1000.000000000000000 ) ;
#3719=ORIENTED_EDGE ( 'NONE', *, *, #7379, .T. ) ;
#3722=CARTESIAN_POINT ( 'NONE',  ( -10.19839929293505776, 1.706249999044084698, -24.62111388750000174 ) ) ;
#3723=CARTESIAN_POINT ( 'NONE',  ( -10.35533905932739174, 4.687500000000000888, 24.99999999999999289 ) ) ;
#3724=( NAMED_UNIT ( * ) SI_UNIT ( $, .STERADIAN. ) SOLID_ANGLE_UNIT ( ) );
#3725=( BOUNDED_CURVE ( )  B_SPLINE_CURVE ( 2, ( #6259, #7860, #1225, #5322, #3762, #285, #3648, #9668, #2751, #5381, #7032, #5266, #10498, #7139, #10392, #2094, #8738, #5470, #4375, #7739, #6925, #10282, #6095, #9455, #1887, #8619, #10660, #1483, #5526, #10705, #9927, #2305, #8109, #9869, #7227, #8013, #442, #4658, #5686, #4810, #1421, #601, #6510, #4866, #8991, #4754, #8210, #2145, #4706, #651, #4028, #543, #5579, #8936, #8169, #9719, #7381, #2199, #3979, #3170, #3069, #3809, #5632, #7182, #10760, #7329, #1325, #3115, #9053, #2361, #6565, #2956, #10547, #5739, #3921, #1370, #2246, #1276, #6361, #10602, #8054 ),
 .UNSPECIFIED., .F., .F. ) 
 B_SPLINE_CURVE_WITH_KNOTS ( ( 3, 2, 2, 2, 2, 2, 2, 2, 2, 2, 2, 2, 2, 2, 2, 2, 2, 2, 2, 2, 2, 2, 2, 2, 2, 2, 2, 2, 2, 2, 2, 2, 2, 2, 2, 2, 2, 2, 2, 2, 3 ),
 ( 0.000000000000000000, 0.02500000000000000139, 0.05000000000000000278, 0.07499999999999999722, 0.1000000000000000056, 0.1250000000000000000, 0.1499999999999999944, 0.1749999999999999889, 0.2000000000000000111, 0.2250000000000000056, 0.2500000000000000000, 0.2750000000000000222, 0.2999999999999999889, 0.3250000000000000111, 0.3499999999999999778, 0.3750000000000000000, 0.4000000000000000222, 0.4249999999999999889, 0.4500000000000000111, 0.4749999999999999778, 0.5000000000000000000, 0.5250000000000000222, 0.5500000000000000444, 0.5749999999999999556, 0.5999999999999999778, 0.6250000000000000000, 0.6500000000000000222, 0.6750000000000000444, 0.6999999999999999556, 0.7249999999999999778, 0.7500000000000000000, 0.7750000000000000222, 0.8000000000000000444, 0.8249999999999999556, 0.8499999999999999778, 0.8750000000000000000, 0.9000000000000000222, 0.9250000000000000444, 0.9499999999999999556, 0.9749999999999999778, 1.000000000000000000 ),
 .UNSPECIFIED. ) 
 CURVE ( )  GEOMETRIC_REPRESENTATION_ITEM ( )  RATIONAL_B_SPLINE_CURVE ( ( 1.000000000000000000, 0.9238795325112867385, 1.000000000000000000, 0.9238795325112867385, 1.000000000000000000, 0.9238795325112867385, 1.000000000000000000, 0.9238795325112867385, 1.000000000000000000, 0.9238795325112867385, 1.000000000000000000, 0.9238795325112867385, 1.000000000000000000, 0.9238795325112867385, 1.000000000000000000, 0.9238795325112867385, 1.000000000000000000, 0.9238795325112867385, 1.000000000000000000, 0.9238795325112867385, 1.000000000000000000, 0.9238795325112867385, 1.000000000000000000, 0.9238795325112867385, 1.000000000000000000, 0.9238795325112867385, 1.000000000000000000, 0.9238795325112867385, 1.000000000000000000, 0.9238795325112867385, 1.000000000000000000, 0.9238795325112867385, 1.000000000000000000, 0.9238795325112867385, 1.000000000000000000, 0.9238795325112867385, 1.000000000000000000, 0.9238795325112867385, 1.000000000000000000, 0.9238795325112867385, 1.000000000000000000, 0.9238795325112867385, 1.000000000000000000, 0.9238795325112867385, 1.000000000000000000, 0.9238795325112867385, 1.000000000000000000, 0.9238795325112867385, 1.000000000000000000, 0.9238795325112867385, 1.000000000000000000, 0.9238795325112867385, 1.000000000000000000, 0.9238795325112867385, 1.000000000000000000, 0.9238795325112867385, 1.000000000000000000, 0.9238795325112867385, 1.000000000000000000, 0.9238795325112867385, 1.000000000000000000, 0.9238795325112867385, 1.000000000000000000, 0.9238795325112867385, 1.000000000000000000, 0.9238795325112867385, 1.000000000000000000, 0.9238795325112867385, 1.000000000000000000, 0.9238795325112867385, 1.000000000000000000, 0.9238795325112867385, 1.000000000000000000, 0.9238795325112867385, 1.000000000000000000, 0.9238795325112867385, 1.000000000000000000, 0.9238795325112867385, 1.000000000000000000, 0.9238795325112867385, 1.000000000000000000 ) ) 
 REPRESENTATION_ITEM ( '' )  );
#3727=CARTESIAN_POINT ( 'NONE',  ( -19.75000000000000000, -0.001000000000001000089, 2.108281996628241301E-13 ) ) ;
#3728=DIRECTION ( 'NONE',  ( 0.000000000000000000, 1.000000000000000000, 0.000000000000000000 ) ) ;
#3733=DIRECTION ( 'NONE',  ( 0.000000000000000000, 1.000000000000000000, 0.000000000000000000 ) ) ;
#3734=VERTEX_POINT ( 'NONE', #722 ) ;
#3735=DIRECTION ( 'NONE',  ( 0.000000000000000000, 0.000000000000000000, -1.000000000000000000 ) ) ;
#3738=DIRECTION ( 'NONE',  ( -0.000000000000000000, 1.000000000000000000, -0.000000000000000000 ) ) ;
#3739=CIRCLE ( 'NONE', #918, 2.999999999999996891 ) ;
#3750=ADVANCED_FACE ( 'NONE', ( #8279 ), #1547, .F. ) ;
#3752=AXIS2_PLACEMENT_3D ( 'NONE', #9851, #5614, #7214 ) ;
#3755=EDGE_CURVE ( 'NONE', #3125, #7345, #5643, .T. ) ;
#3758=CIRCLE ( 'NONE', #3575, 2.999999999999999112 ) ;
#3762=CARTESIAN_POINT ( 'NONE',  ( 1.507608415688466075E-15, 0.6437499990440845865, -24.62111388750000174 ) ) ;
#3764=DIRECTION ( 'NONE',  ( -0.000000000000000000, 1.000000000000000000, -0.000000000000000000 ) ) ;
#3767=AXIS2_PLACEMENT_3D ( 'NONE', #2604, #2489, #4171 ) ;
#3769=CARTESIAN_POINT ( 'NONE',  ( 25.00000000000000000, 2.612499998088169129, 0.000000000000000000 ) ) ;
#3775=CIRCLE ( 'NONE', #6958, 2.999999999999999112 ) ;
#3777=DIRECTION ( 'NONE',  ( -0.000000000000000000, -1.000000000000000000, -0.000000000000000000 ) ) ;
#3779=CARTESIAN_POINT ( 'NONE',  ( 17.40975659021752620, 2.268749999044084475, 17.40975659021753330 ) ) ;
#3781=CARTESIAN_POINT ( 'NONE',  ( 1.530808498934191521E-15, 2.250000000000000444, -25.00000000000000000 ) ) ;
#3784=CARTESIAN_POINT ( 'NONE',  ( -25.00000000000000000, 1.112499998088169351, -3.061616997868383043E-15 ) ) ;
#3785=DIRECTION ( 'NONE',  ( 0.8660254037844407060, 0.4999999999999965583, -0.000000000000000000 ) ) ;
#3790=ORIENTED_EDGE ( 'NONE', *, *, #9500, .T. ) ;
#3792=PLANE ( 'NONE',  #7831 ) ;
#3798=ORIENTED_EDGE ( 'NONE', *, *, #7234, .F. ) ;
#3801=DIRECTION ( 'NONE',  ( 0.8660254037844417052, 0.000000000000000000, 0.4999999999999947820 ) ) ;
#3809=CARTESIAN_POINT ( 'NONE',  ( 10.19839929293506486, 4.206249999044083587, 24.62111388749999819 ) ) ;
#3810=ORIENTED_EDGE ( 'NONE', *, *, #5114, .T. ) ;
#3817=EDGE_CURVE ( 'NONE', #7899, #4897, #9009, .T. ) ;
#3820=ORIENTED_EDGE ( 'NONE', *, *, #6894, .F. ) ;
#3821=VERTEX_POINT ( 'NONE', #9007 ) ;
#3822=ORIENTED_EDGE ( 'NONE', *, *, #7885, .T. ) ;
#3823=EDGE_CURVE ( 'NONE', #9950, #9951, #4946, .T. ) ;
#3826=CARTESIAN_POINT ( 'NONE',  ( 24.62111388750000174, 4.456249999044085364, -10.19839929293505776 ) ) ;
#3827=EDGE_LOOP ( 'NONE', ( #10899, #3719, #7995, #7315 ) ) ;
#3828=CARTESIAN_POINT ( 'NONE',  ( -4.592425496802574367E-15, 1.750000000000000000, 25.00000000000000000 ) ) ;
#3833=EDGE_CURVE ( 'NONE', #2200, #2242, #7377, .T. ) ;
#3835=VERTEX_POINT ( 'NONE', #1837 ) ;
#3836=ORIENTED_EDGE ( 'NONE', *, *, #8352, .T. ) ;
#3837=EDGE_CURVE ( 'NONE', #3225, #7963, #7423, .T. ) ;
#3838=CARTESIAN_POINT ( 'NONE',  ( -25.00000000000000000, 4.437500000000001776, -10.35533905932738108 ) ) ;
#3842=CARTESIAN_POINT ( 'NONE',  ( -15.60400172474278158, 28.00000000000000000, -12.47307621135316680 ) ) ;
#3846=EDGE_CURVE ( 'NONE', #963, #849, #10410, .T. ) ;
#3849=EDGE_CURVE ( 'NONE', #7097, #10741, #5670, .T. ) ;
#3851=AXIS2_PLACEMENT_3D ( 'NONE', #5438, #2165, #10565 ) ;
#3853=DIRECTION ( 'NONE',  ( -0.000000000000000000, -1.000000000000000000, -0.000000000000000000 ) ) ;
#3855=DIRECTION ( 'NONE',  ( -0.000000000000000000, 1.000000000000000000, 0.000000000000000000 ) ) ;
#3856=CARTESIAN_POINT ( 'NONE',  ( -12.47307621135311351, -0.001000000000001000089, 15.60400172474282599 ) ) ;
#3858=CIRCLE ( 'NONE', #1926, 2.999999999999999112 ) ;
#3861=LINE ( 'NONE', #1481, #4793 ) ;
#3863=LINE ( 'NONE', #3013, #6234 ) ;
#3868=ORIENTED_EDGE ( 'NONE', *, *, #2469, .T. ) ;
#3875=CARTESIAN_POINT ( 'NONE',  ( 17.40975659021752975, 1.518749999044084698, -17.40975659021752975 ) ) ;
#3878=CARTESIAN_POINT ( 'NONE',  ( -25.00000000000000000, 2.437500000000000444, -10.35533905932738108 ) ) ;
#3880=CARTESIAN_POINT ( 'NONE',  ( -17.67766952966369232, 1.237499998088169129, 17.67766952966368876 ) ) ;
#3883=AXIS2_PLACEMENT_3D ( 'NONE', #1824, #10097, #6086 ) ;
#3885=ADVANCED_FACE ( 'NONE', ( #1065 ), #10284, .F. ) ;
#3887=ORIENTED_EDGE ( 'NONE', *, *, #2012, .F. ) ;
#3891=AXIS2_PLACEMENT_3D ( 'NONE', #6127, #1750, #1983 ) ;
#3892=AXIS2_PLACEMENT_3D ( 'NONE', #6694, #888, #831 ) ;
#3895=EDGE_CURVE ( 'NONE', #4070, #1064, #5982, .T. ) ;
#3897=CYLINDRICAL_SURFACE ( 'NONE', #5003, 2.999999999999997335 ) ;
#3898=VERTEX_POINT ( 'NONE', #58 ) ;
#3902=DIRECTION ( 'NONE',  ( 0.5000000000000009992, 0.000000000000000000, 0.8660254037844380415 ) ) ;
#3905=AXIS2_PLACEMENT_3D ( 'NONE', #3112, #5684, #2511 ) ;
#3907=ORIENTED_EDGE ( 'NONE', *, *, #8828, .T. ) ;
#3908=EDGE_LOOP ( 'NONE', ( #3091, #1132, #7338, #10849 ) ) ;
#3910=DIRECTION ( 'NONE',  ( -0.000000000000000000, -1.000000000000000000, -0.000000000000000000 ) ) ;
#3914=ADVANCED_FACE ( 'NONE', ( #3595 ), #6983, .F. ) ;
#3916=ADVANCED_FACE ( 'NONE', ( #3417 ), #8503, .F. ) ;
#3918=VERTEX_POINT ( 'NONE', #112 ) ;
#3921=CARTESIAN_POINT ( 'NONE',  ( -17.40975659021753330, 5.018749999044084475, 17.40975659021752975 ) ) ;
#3924=CARTESIAN_POINT ( 'NONE',  ( 24.81055694375000087, 5.109374999522041882, 0.000000000000000000 ) ) ;
#3925=CARTESIAN_POINT ( 'NONE',  ( 7.875000000000019540, 25.00000000000000000, 13.63990010960489840 ) ) ;
#3926=EDGE_CURVE ( 'NONE', #10105, #3577, #9269, .T. ) ;
#3927=ORIENTED_EDGE ( 'NONE', *, *, #2196, .F. ) ;
#3929=CARTESIAN_POINT ( 'NONE',  ( 10.19839929293506486, 3.031249999044084653, 24.62111388749999819 ) ) ;
#3930=VECTOR ( 'NONE', #8719, 1000.000000000000000 ) ;
#3931=VERTEX_POINT ( 'NONE', #444 ) ;
#3932=ORIENTED_EDGE ( 'NONE', *, *, #1696, .T. ) ;
#3933=AXIS2_PLACEMENT_3D ( 'NONE', #10025, #2447, #9301 ) ;
#3939=CARTESIAN_POINT ( 'NONE',  ( 24.62111388749999463, 1.331249999044084475, 10.19839929293507730 ) ) ;
#3940=DIRECTION ( 'NONE',  ( 0.000000000000000000, 1.000000000000000000, 0.000000000000000000 ) ) ;
#3941=CARTESIAN_POINT ( 'NONE',  ( 0.000000000000000000, 85.00000000000000000, 0.000000000000000000 ) ) ;
#3945=CIRCLE ( 'NONE', #5371, 2.999999999999998224 ) ;
#3946=DIRECTION ( 'NONE',  ( 0.000000000000000000, 0.000000000000000000, -1.000000000000000000 ) ) ;
#3952=VECTOR ( 'NONE', #1864, 1000.000000000000000 ) ;
#3955=CARTESIAN_POINT ( 'NONE',  ( -15.74999999999997158, 28.00000000000000000, 3.000000000000165645 ) ) ;
#3957=CARTESIAN_POINT ( 'NONE',  ( 1.530808498934191521E-15, 4.862499998088169129, -25.00000000000000000 ) ) ;
#3959=CARTESIAN_POINT ( 'NONE',  ( 15.60400172474269453, 28.00000000000000000, 12.47307621135327693 ) ) ;
#3960=DIRECTION ( 'NONE',  ( 0.000000000000000000, 1.000000000000000000, 0.000000000000000000 ) ) ;
#3962=EDGE_CURVE ( 'NONE', #1334, #857, #4661, .T. ) ;
#3964=VERTEX_POINT ( 'NONE', #10394 ) ;
#3970=DIRECTION ( 'NONE',  ( 0.000000000000000000, 1.000000000000000000, 0.000000000000000000 ) ) ;
#3971=CARTESIAN_POINT ( 'NONE',  ( 10.35533905932737930, 0.1874999999999999722, -25.00000000000000000 ) ) ;
#3974=VERTEX_POINT ( 'NONE', #8740 ) ;
#3975=EDGE_LOOP ( 'NONE', ( #9001, #7339, #10556, #6118, #10077, #10933 ) ) ;
#3977=LINE ( 'NONE', #7328, #7413 ) ;
#3979=CARTESIAN_POINT ( 'NONE',  ( -17.40975659021753330, 4.018749999044084475, 17.40975659021752975 ) ) ;
#3980=ORIENTED_EDGE ( 'NONE', *, *, #10904, .F. ) ;
#3986=EDGE_LOOP ( 'NONE', ( #5307, #807, #8021, #891, #9823 ) ) ;
#3992=CARTESIAN_POINT ( 'NONE',  ( -24.62111388750000174, 1.656249999044084431, -10.19839929293506131 ) ) ;
#3993=ORIENTED_EDGE ( 'NONE', *, *, #6744, .F. ) ;
#3994=DIRECTION ( 'NONE',  ( 1.000000000000000000, 0.000000000000000000, -1.069128445102650095E-14 ) ) ;
#3995=LINE ( 'NONE', #837, #3497 ) ;
#3996=CARTESIAN_POINT ( 'NONE',  ( 17.67766952966368521, 1.487499998088169129, 17.67766952966369232 ) ) ;
#4003=CARTESIAN_POINT ( 'NONE',  ( 1.507608415688466075E-15, 0.4687499990440845421, -24.62111388750000174 ) ) ;
#4009=CARTESIAN_POINT ( 'NONE',  ( 9.875000000000023093, 28.00000000000000000, 17.10400172474264835 ) ) ;
#4012=EDGE_LOOP ( 'NONE', ( #4268, #2607, #2311, #8044, #8095 ) ) ;
#4014=ORIENTED_EDGE ( 'NONE', *, *, #2336, .T. ) ;
#4016=CARTESIAN_POINT ( 'NONE',  ( -9.874999999999777955, 25.00000000000000000, 20.10400172474279401 ) ) ;
#4023=ADVANCED_FACE ( 'NONE', ( #5426 ), #8838, .T. ) ;
#4025=EDGE_LOOP ( 'NONE', ( #7691, #6152, #7634, #10615 ) ) ;
#4026=DIRECTION ( 'NONE',  ( 0.000000000000000000, 1.000000000000000000, -0.000000000000000000 ) ) ;
#4027=VECTOR ( 'NONE', #6542, 1000.000000000000000 ) ;
#4028=CARTESIAN_POINT ( 'NONE',  ( 17.40975659021752975, 3.518749999044084920, -17.40975659021752975 ) ) ;
#4035=AXIS2_PLACEMENT_3D ( 'NONE', #5166, #4332, #8515 ) ;
#4037=CARTESIAN_POINT ( 'NONE',  ( -24.62111388750000174, 1.718749999044084431, -3.015216831376932151E-15 ) ) ;
#4038=ORIENTED_EDGE ( 'NONE', *, *, #9277, .T. ) ;
#4039=ADVANCED_FACE ( 'NONE', ( #3708 ), #4609, .F. ) ;
#4044=CARTESIAN_POINT ( 'NONE',  ( -24.62111388750000884, 0.7812499990440845421, 10.19839929293505421 ) ) ;
#4048=DIRECTION ( 'NONE',  ( -0.000000000000000000, 1.000000000000000000, 0.000000000000000000 ) ) ;
#4049=CARTESIAN_POINT ( 'NONE',  ( -3.957930336368489021E-15, 25.00000000000000000, -19.75000000000000000 ) ) ;
#4053=ORIENTED_EDGE ( 'NONE', *, *, #5144, .T. ) ;
#4056=CARTESIAN_POINT ( 'NONE',  ( 17.40975659021752620, 1.093749999044084653, 17.40975659021753330 ) ) ;
#4059=AXIS2_PLACEMENT_3D ( 'NONE', #9530, #1086, #9586 ) ;
#4065=EDGE_LOOP ( 'NONE', ( #2508, #4424, #10294, #4228, #7222 ) ) ;
#4067=ORIENTED_EDGE ( 'NONE', *, *, #6130, .F. ) ;
#4069=CIRCLE ( 'NONE', #703, 2.999999999999999112 ) ;
#4070=VERTEX_POINT ( 'NONE', #6306 ) ;
#4072=LINE ( 'NONE', #7218, #9936 ) ;
#4073=CARTESIAN_POINT ( 'NONE',  ( 1.530808498934191521E-15, 4.862499998088169129, -25.00000000000000000 ) ) ;
#4074=VECTOR ( 'NONE', #3777, 1000.000000000000000 ) ;
#4077=CARTESIAN_POINT ( 'NONE',  ( -15.75000000000003553, 28.00000000000000000, -2.999999999999832578 ) ) ;
#4087=VERTEX_POINT ( 'NONE', #4708 ) ;
#4089=CARTESIAN_POINT ( 'NONE',  ( 24.62111388750000174, 2.218749999044084653, 0.000000000000000000 ) ) ;
#4091=ORIENTED_EDGE ( 'NONE', *, *, #2357, .F. ) ;
#4092=VECTOR ( 'NONE', #3785, 1000.000000000000114 ) ;
#4095=ORIENTED_EDGE ( 'NONE', *, *, #1153, .T. ) ;
#4098=CARTESIAN_POINT ( 'NONE',  ( 12.47307621135322186, 28.00000000000000000, -15.60400172474273717 ) ) ;
#4099=CARTESIAN_POINT ( 'NONE',  ( -17.40975659021752975, 2.593749999044084653, -17.40975659021752975 ) ) ;
#4100=VERTEX_POINT ( 'NONE', #7502 ) ;
#4101=DIRECTION ( 'NONE',  ( 1.069128445102650095E-14, 0.000000000000000000, 1.000000000000000000 ) ) ;
#4102=EDGE_CURVE ( 'NONE', #7345, #1671, #3171, .T. ) ;
#4104=CARTESIAN_POINT ( 'NONE',  ( -17.67766952966369232, 2.237499998088169573, 17.67766952966368876 ) ) ;
#4109=AXIS2_PLACEMENT_3D ( 'NONE', #7729, #881, #7792 ) ;
#4119=CARTESIAN_POINT ( 'NONE',  ( 7.276923788646707969, 28.00000000000000000, 18.60400172474265190 ) ) ;
#4120=DIRECTION ( 'NONE',  ( 0.000000000000000000, -0.000000000000000000, 1.000000000000000000 ) ) ;
#4128=ORIENTED_EDGE ( 'NONE', *, *, #8947, .T. ) ;
#4133=DIRECTION ( 'NONE',  ( 0.000000000000000000, 0.000000000000000000, 1.000000000000000000 ) ) ;
#4134=DIRECTION ( 'NONE',  ( 0.8660254037844399289, 0.000000000000000000, 0.4999999999999978351 ) ) ;
#4135=CARTESIAN_POINT ( 'NONE',  ( 0.000000000000000000, 28.00000000000000000, -10.50000000000000000 ) ) ;
#4136=ORIENTED_EDGE ( 'NONE', *, *, #9583, .T. ) ;
#4147=CARTESIAN_POINT ( 'NONE',  ( 10.19839929293506486, 1.031249999044084653, 24.62111388749999819 ) ) ;
#4150=CARTESIAN_POINT ( 'NONE',  ( 0.000000000000000000, 25.00000000000000000, -25.00000000000000000 ) ) ;
#4151=CARTESIAN_POINT ( 'NONE',  ( -10.19839929293507552, 1.906249999044084431, 24.62111388749999463 ) ) ;
#4154=CARTESIAN_POINT ( 'NONE',  ( 3.957930336368489021E-15, 28.00000000000000000, 19.75000000000000000 ) ) ;
#4157=DIRECTION ( 'NONE',  ( 1.000000000000000000, 0.000000000000000000, -3.708321773340234242E-15 ) ) ;
#4160=DIRECTION ( 'NONE',  ( -0.4999999999999887312, 0.000000000000000000, 0.8660254037844451469 ) ) ;
#4162=ORIENTED_EDGE ( 'NONE', *, *, #106, .T. ) ;
#4164=CARTESIAN_POINT ( 'NONE',  ( 24.99999999999999289, 5.549999998088169129, 10.35533905932739529 ) ) ;
#4165=CARTESIAN_POINT ( 'NONE',  ( 10.19839929293505953, 1.406249999044084653, -24.62111388750000174 ) ) ;
#4171=DIRECTION ( 'NONE',  ( 0.000000000000000000, 0.000000000000000000, 1.000000000000000000 ) ) ;
#4178=CARTESIAN_POINT ( 'NONE',  ( -10.47307621135341904, 28.00000000000000000, -12.13990010960482557 ) ) ;
#4188=EDGE_LOOP ( 'NONE', ( #9158, #4638, #9295, #418 ) ) ;
#4189=DIRECTION ( 'NONE',  ( 2.168404344971010347E-16, 0.000000000000000000, 1.000000000000000000 ) ) ;
#4191=CARTESIAN_POINT ( 'NONE',  ( 0.000000000000000000, 85.00000000000000000, -25.00000000000000000 ) ) ;
#4192=AXIS2_PLACEMENT_3D ( 'NONE', #10931, #2512, #5904 ) ;
#4194=CARTESIAN_POINT ( 'NONE',  ( -4.522825247065398226E-15, 3.968749999044084209, 24.62111388750000174 ) ) ;
#4196=ORIENTED_EDGE ( 'NONE', *, *, #7843, .F. ) ;
#4199=CARTESIAN_POINT ( 'NONE',  ( 19.75000000000001066, 25.00000000000000000, 2.999999999999927613 ) ) ;
#4200=CARTESIAN_POINT ( 'NONE',  ( -24.62111388750000174, 2.656249999044085097, -10.19839929293506131 ) ) ;
#4202=ORIENTED_EDGE ( 'NONE', *, *, #3076, .F. ) ;
#4203=CARTESIAN_POINT ( 'NONE',  ( -10.35533905932739174, 3.687500000000000444, 24.99999999999999289 ) ) ;
#4205=DIRECTION ( 'NONE',  ( -0.000000000000000000, -1.000000000000000000, -0.000000000000000000 ) ) ;
#4206=CARTESIAN_POINT ( 'NONE',  ( 3.061616997868383043E-15, 85.00000000000000000, 25.00000000000000000 ) ) ;
#4207=CARTESIAN_POINT ( 'NONE',  ( 0.000000000000000000, 0.000000000000000000, -28.00000000000000000 ) ) ;
#4210=ORIENTED_EDGE ( 'NONE', *, *, #8400, .F. ) ;
#4214=CARTESIAN_POINT ( 'NONE',  ( -10.19839929293507552, 2.081249999044084475, 24.62111388749999463 ) ) ;
#4215=CARTESIAN_POINT ( 'NONE',  ( 24.62111388749999463, 2.156249999044085097, 10.19839929293507730 ) ) ;
#4226=ADVANCED_FACE ( 'NONE', ( #5581 ), #1485, .F. ) ;
#4227=EDGE_CURVE ( 'NONE', #8104, #10668, #8938, .T. ) ;
#4228=ORIENTED_EDGE ( 'NONE', *, *, #9500, .F. ) ;
#4230=AXIS2_PLACEMENT_3D ( 'NONE', #6326, #2112, #5493 ) ;
#4231=CARTESIAN_POINT ( 'NONE',  ( -10.47307621135315792, -0.001000000000001000089, 12.13990010960504762 ) ) ;
#4233=DIRECTION ( 'NONE',  ( -0.8660254037844328234, 0.000000000000000000, 0.5000000000000098810 ) ) ;
#4234=EDGE_CURVE ( 'NONE', #5714, #3931, #6465, .T. ) ;
#4236=CARTESIAN_POINT ( 'NONE',  ( 12.13990010960493748, 28.00000000000000000, 10.47307621135328759 ) ) ;
#4237=DIRECTION ( 'NONE',  ( 0.000000000000000000, 0.000000000000000000, 1.000000000000000000 ) ) ;
#4238=VECTOR ( 'NONE', #7283, 1000.000000000000114 ) ;
#4245=CIRCLE ( 'NONE', #5663, 2.999999999999997335 ) ;
#4250=CARTESIAN_POINT ( 'NONE',  ( 3.429011037612589276E-15, 85.00000000000000000, 28.00000000000000000 ) ) ;
#4251=CYLINDRICAL_SURFACE ( 'NONE', #7203, 7.500000000000000888 ) ;
#4253=ORIENTED_EDGE ( 'NONE', *, *, #9275, .T. ) ;
#4258=LINE ( 'NONE', #55, #1534 ) ;
#4261=FACE_OUTER_BOUND ( 'NONE', #471, .T. ) ;
#4265=VECTOR ( 'NONE', #8526, 1000.000000000000000 ) ;
#4266=VERTEX_POINT ( 'NONE', #220 ) ;
#4268=ORIENTED_EDGE ( 'NONE', *, *, #3060, .F. ) ;
#4269=ORIENTED_EDGE ( 'NONE', *, *, #3634, .T. ) ;
#4270=DIRECTION ( 'NONE',  ( 0.000000000000000000, 0.000000000000000000, -1.000000000000000000 ) ) ;
#4274=CARTESIAN_POINT ( 'NONE',  ( 24.62111388750000174, 1.456249999044084475, -10.19839929293505776 ) ) ;
#4275=CARTESIAN_POINT ( 'NONE',  ( 25.00000000000000000, 1.000000000000000000, 0.000000000000000000 ) ) ;
#4276=LINE ( 'NONE', #3370, #5088 ) ;
#4286=CIRCLE ( 'NONE', #2854, 2.999999999999996447 ) ;
#4288=EDGE_LOOP ( 'NONE', ( #6425, #141, #7123, #8211 ) ) ;
#4289=CIRCLE ( 'NONE', #940, 2.999999999999998668 ) ;
#4296=DIRECTION ( 'NONE',  ( -0.8660254037844344888, 0.000000000000000000, 0.5000000000000074385 ) ) ;
#4297=EDGE_CURVE ( 'NONE', #9541, #3898, #5655, .T. ) ;
#4298=CARTESIAN_POINT ( 'NONE',  ( 3.000000000000000888, -0.001000000000001000089, 15.75000000000000355 ) ) ;
#4299=CARTESIAN_POINT ( 'NONE',  ( 9.874999999999895195, 25.00000000000000000, -17.10400172474272651 ) ) ;
#4302=EDGE_CURVE ( 'NONE', #5017, #5745, #1053, .T. ) ;
#4308=CARTESIAN_POINT ( 'NONE',  ( -12.47307621135311351, 25.00000000000000000, 15.60400172474282599 ) ) ;
#4310=DIRECTION ( 'NONE',  ( -0.000000000000000000, -1.000000000000000000, -0.000000000000000000 ) ) ;
#4312=PLANE ( 'NONE',  #4109 ) ;
#4315=EDGE_CURVE ( 'NONE', #3378, #8379, #3403, .T. ) ;
#4320=DIRECTION ( 'NONE',  ( 0.000000000000000000, 0.000000000000000000, -1.000000000000000000 ) ) ;
#4321=VERTEX_POINT ( 'NONE', #9380 ) ;
#4322=CARTESIAN_POINT ( 'NONE',  ( 9.874999999999895195, -0.001000000000001000089, -17.10400172474272651 ) ) ;
#4323=CYLINDRICAL_SURFACE ( 'NONE', #8333, 25.00000000000000000 ) ;
#4324=DIRECTION ( 'NONE',  ( -0.000000000000000000, 1.000000000000000000, -0.000000000000000000 ) ) ;
#4326=LINE ( 'NONE', #117, #734 ) ;
#4328=ORIENTED_EDGE ( 'NONE', *, *, #10595, .T. ) ;
#4331=ORIENTED_EDGE ( 'NONE', *, *, #7205, .F. ) ;
#4332=DIRECTION ( 'NONE',  ( -0.000000000000000000, -1.000000000000000000, -0.000000000000000000 ) ) ;
#4334=CARTESIAN_POINT ( 'NONE',  ( -17.40975659021752975, 0.7687499990440846975, -17.40975659021752975 ) ) ;
#4335=CARTESIAN_POINT ( 'NONE',  ( -17.40975659021752975, 1.768749999044084475, -17.40975659021752975 ) ) ;
#4336=CARTESIAN_POINT ( 'NONE',  ( -24.62111388750000174, 2.718749999044084653, -3.015216831376932151E-15 ) ) ;
#4337=CARTESIAN_POINT ( 'NONE',  ( -17.67766952966369232, 3.237499998088169573, 17.67766952966368876 ) ) ;
#4339=CARTESIAN_POINT ( 'NONE',  ( 0.000000000000000000, 85.00000000000000000, 0.000000000000000000 ) ) ;
#4341=EDGE_LOOP ( 'NONE', ( #9456, #8007, #10190, #7131 ) ) ;
#4342=ORIENTED_EDGE ( 'NONE', *, *, #5575, .F. ) ;
#4343=EDGE_LOOP ( 'NONE', ( #2443, #10847, #9278, #9669 ) ) ;
#4348=CARTESIAN_POINT ( 'NONE',  ( -7.276923788646840308, -0.001000000000001000089, -18.60400172474260216 ) ) ;
#4349=DIRECTION ( 'NONE',  ( 1.156482317317872514E-15, 0.000000000000000000, 1.000000000000000000 ) ) ;
#4350=DIRECTION ( 'NONE',  ( 0.000000000000000000, 0.000000000000000000, 1.000000000000000000 ) ) ;
#4352=CARTESIAN_POINT ( 'NONE',  ( -15.60400172474251868, 25.00000000000000000, 12.47307621135349720 ) ) ;
#4354=CARTESIAN_POINT ( 'NONE',  ( 17.40975659021752620, 4.268749999044084475, 17.40975659021753330 ) ) ;
#4356=EDGE_LOOP ( 'NONE', ( #4728, #608 ) ) ;
#4359=CARTESIAN_POINT ( 'NONE',  ( -17.67766952966368876, 3.987499998088168685, -17.67766952966369232 ) ) ;
#4366=CARTESIAN_POINT ( 'NONE',  ( -24.62111388750000884, 4.781249999044083765, 10.19839929293505421 ) ) ;
#4367=ADVANCED_FACE ( 'NONE', ( #3581 ), #1761, .F. ) ;
#4374=DIRECTION ( 'NONE',  ( 0.000000000000000000, 1.000000000000000000, -0.000000000000000000 ) ) ;
#4375=CARTESIAN_POINT ( 'NONE',  ( 17.40975659021752975, 1.518749999044084698, -17.40975659021752975 ) ) ;
#4377=DIRECTION ( 'NONE',  ( 0.000000000000000000, 0.000000000000000000, 1.000000000000000000 ) ) ;
#4383=DIRECTION ( 'NONE',  ( -0.000000000000000000, -1.000000000000000000, -0.000000000000000000 ) ) ;
#4385=EDGE_CURVE ( 'NONE', #9894, #4100, #4428, .T. ) ;
#4386=EDGE_LOOP ( 'NONE', ( #4513, #8036, #2182, #8266 ) ) ;
#4391=CARTESIAN_POINT ( 'NONE',  ( -24.62111388750000174, 0.8937499990440845865, -3.015216831376932151E-15 ) ) ;
#4392=CARTESIAN_POINT ( 'NONE',  ( -25.00000000000000000, 5.049999998088170017, -10.35533905932738108 ) ) ;
#4393=CARTESIAN_POINT ( 'NONE',  ( 10.19839929293506486, 5.031249999044083765, 24.62111388749999819 ) ) ;
#4401=CARTESIAN_POINT ( 'NONE',  ( 15.60400172474260927, -0.001000000000001000089, -12.47307621135339062 ) ) ;
#4403=AXIS2_PLACEMENT_3D ( 'NONE', #5057, #1675, #9467 ) ;
#4405=DIRECTION ( 'NONE',  ( -0.8660254037844398178, 0.000000000000000000, -0.4999999999999977796 ) ) ;
#4406=ORIENTED_EDGE ( 'NONE', *, *, #936, .T. ) ;
#4408=EDGE_LOOP ( 'NONE', ( #3394, #7087, #7392, #923, #99, #981, #10037, #5414, #3798, #4967, #730, #3927, #9688, #8830 ) ) ;
#4409=DIRECTION ( 'NONE',  ( 0.8660254037844362651, 0.000000000000000000, -0.5000000000000042188 ) ) ;
#4411=DIRECTION ( 'NONE',  ( 1.000000000000000000, 0.000000000000000000, -3.491481338843131383E-15 ) ) ;
#4412=DIRECTION ( 'NONE',  ( 0.000000000000000000, 0.000000000000000000, 1.000000000000000000 ) ) ;
#4415=DIRECTION ( 'NONE',  ( -0.000000000000000000, -1.000000000000000000, -0.000000000000000000 ) ) ;
#4417=CARTESIAN_POINT ( 'NONE',  ( -4.592425496802574367E-15, 4.362499998088169129, 25.00000000000000000 ) ) ;
#4421=CARTESIAN_POINT ( 'NONE',  ( 25.00000000000000000, 5.612499998088169129, 0.000000000000000000 ) ) ;
#4424=ORIENTED_EDGE ( 'NONE', *, *, #1390, .F. ) ;
#4427=FACE_OUTER_BOUND ( 'NONE', #3908, .T. ) ;
#4428=CIRCLE ( 'NONE', #10584, 2.999999999999996447 ) ;
#4430=DIRECTION ( 'NONE',  ( 0.000000000000000000, 1.000000000000000000, 0.000000000000000000 ) ) ;
#4431=CARTESIAN_POINT ( 'NONE',  ( -10.19839929293505776, 4.531249999044084653, -24.62111388750000174 ) ) ;
#4437=CARTESIAN_POINT ( 'NONE',  ( -10.19839929293505776, 4.531249999044084653, -24.62111388750000174 ) ) ;
#4443=FACE_BOUND ( 'NONE', #7709, .T. ) ;
#4444=CARTESIAN_POINT ( 'NONE',  ( -4.592425496802574367E-15, 1.362499998088169129, 25.00000000000000000 ) ) ;
#4449=ADVANCED_FACE ( 'NONE', ( #5083 ), #876, .F. ) ;
#4451=ORIENTED_EDGE ( 'NONE', *, *, #7042, .F. ) ;
#4452=EDGE_CURVE ( 'NONE', #7447, #2032, #2986, .T. ) ;
#4455=CARTESIAN_POINT ( 'NONE',  ( 5.276923788646705304, 28.00000000000000000, 15.13990010960490196 ) ) ;
#4456=CARTESIAN_POINT ( 'NONE',  ( 10.35533905932737930, 4.799999998088169129, -25.00000000000000000 ) ) ;
#4457=CARTESIAN_POINT ( 'NONE',  ( 10.19839929293505953, 4.406249999044084653, -24.62111388750000174 ) ) ;
#4458=AXIS2_PLACEMENT_3D ( 'NONE', #9080, #1622, #8241 ) ;
#4460=CARTESIAN_POINT ( 'NONE',  ( 0.000000000000000000, 85.00000000000000000, -25.00000000000000000 ) ) ;
#4461=FACE_BOUND ( 'NONE', #9727, .T. ) ;
#4463=LINE ( 'NONE', #10244, #6212 ) ;
#4465=ADVANCED_FACE ( 'NONE', ( #326 ), #5458, .F. ) ;
#4466=DIRECTION ( 'NONE',  ( -0.000000000000000000, 1.000000000000000000, -0.000000000000000000 ) ) ;
#4470=AXIS2_PLACEMENT_3D ( 'NONE', #10842, #1669, #9116 ) ;
#4473=EDGE_CURVE ( 'NONE', #7275, #9592, #5511, .T. ) ;
#4478=DIRECTION ( 'NONE',  ( 0.000000000000000000, 1.000000000000000000, 0.000000000000000000 ) ) ;
#4480=CARTESIAN_POINT ( 'NONE',  ( 0.000000000000000000, 28.00000000000000000, 0.000000000000000000 ) ) ;
#4481=DIRECTION ( 'NONE',  ( -0.000000000000000000, 1.000000000000000000, -0.000000000000000000 ) ) ;
#4482=CARTESIAN_POINT ( 'NONE',  ( -10.35533905932737575, 1.312500000000000222, -25.00000000000000000 ) ) ;
#4483=CARTESIAN_POINT ( 'NONE',  ( -10.19839929293505776, 4.706249999044084475, -24.62111388750000174 ) ) ;
#4484=VECTOR ( 'NONE', #205, 1000.000000000000000 ) ;
#4487=ORIENTED_EDGE ( 'NONE', *, *, #6647, .F. ) ;
#4490=PRESENTATION_STYLE_ASSIGNMENT (( #3691 ) ) ;
#4492=ORIENTED_EDGE ( 'NONE', *, *, #7670, .T. ) ;
#4497=CARTESIAN_POINT ( 'NONE',  ( -4.592425496802574367E-15, 5.362499998088169129, 25.00000000000000000 ) ) ;
#4499=AXIS2_PLACEMENT_3D ( 'NONE', #101, #2516, #7727 ) ;
#4501=AXIS2_PLACEMENT_3D ( 'NONE', #9485, #7009, #10527 ) ;
#4503=VECTOR ( 'NONE', #2613, 1000.000000000000000 ) ;
#4504=CARTESIAN_POINT ( 'NONE',  ( 7.276923788646575630, 28.00000000000000000, -18.60400172474270875 ) ) ;
#4511=PLANE ( 'NONE',  #6246 ) ;
#4513=ORIENTED_EDGE ( 'NONE', *, *, #4709, .F. ) ;
#4516=CARTESIAN_POINT ( 'NONE',  ( 10.47307621135324496, 28.00000000000000000, -12.13990010960497479 ) ) ;
#4518=CARTESIAN_POINT ( 'NONE',  ( 10.35533905932737930, 0.7999999980881692396, -25.00000000000000000 ) ) ;
#4519=ADVANCED_FACE ( 'NONE', ( #1994 ), #10489, .F. ) ;
#4520=CARTESIAN_POINT ( 'NONE',  ( 25.00000000000000000, 3.612499998088169129, 0.000000000000000000 ) ) ;
#4521=CARTESIAN_POINT ( 'NONE',  ( 10.35533905932737930, 0.1874999999999999722, -25.00000000000000000 ) ) ;
#4524=DIRECTION ( 'NONE',  ( -0.000000000000000000, -1.000000000000000000, -0.000000000000000000 ) ) ;
#4530=ORIENTED_EDGE ( 'NONE', *, *, #130, .F. ) ;
#4534=CARTESIAN_POINT ( 'NONE',  ( -18.60400172474273361, -0.001000000000001000089, -7.276923788646511682 ) ) ;
#4535=ORIENTED_EDGE ( 'NONE', *, *, #1541, .T. ) ;
#4537=DIRECTION ( 'NONE',  ( -0.4999999999999977796, -0.000000000000000000, 0.8660254037844399289 ) ) ;
#4538=FACE_OUTER_BOUND ( 'NONE', #8724, .T. ) ;
#4539=DIRECTION ( 'NONE',  ( 0.000000000000000000, 0.000000000000000000, 1.000000000000000000 ) ) ;
#4544=EDGE_LOOP ( 'NONE', ( #1165, #8722, #4196, #1888 ) ) ;
#4545=FILL_AREA_STYLE ('',( #9795 ) ) ;
#4548=CARTESIAN_POINT ( 'NONE',  ( 15.74999999999999289, 28.00000000000000000, -3.000000000000055955 ) ) ;
#4549=EDGE_CURVE ( 'NONE', #8189, #1816, #7224, .T. ) ;
#4550=DIRECTION ( 'NONE',  ( 0.000000000000000000, 0.000000000000000000, 1.000000000000000000 ) ) ;
#4558=CARTESIAN_POINT ( 'NONE',  ( 15.13990010960492505, 28.00000000000000000, 5.276923788646651126 ) ) ;
#4560=DIRECTION ( 'NONE',  ( 0.000000000000000000, 0.000000000000000000, 1.000000000000000000 ) ) ;
#4562=ORIENTED_EDGE ( 'NONE', *, *, #8080, .T. ) ;
#4568=CARTESIAN_POINT ( 'NONE',  ( 10.19839929293505953, 4.581249999044085364, -24.62111388750000174 ) ) ;
#4569=CARTESIAN_POINT ( 'NONE',  ( -10.35533905932739174, 4.299999998088169129, 24.99999999999999289 ) ) ;
#4570=CARTESIAN_POINT ( 'NONE',  ( 25.00000000000000000, 3.062500000000000000, -10.35533905932737753 ) ) ;
#4571=DIRECTION ( 'NONE',  ( 0.000000000000000000, 0.000000000000000000, 1.000000000000000000 ) ) ;
#4575=DIRECTION ( 'NONE',  ( -0.5000000000000042188, 0.000000000000000000, -0.8660254037844362651 ) ) ;
#4578=ORIENTED_EDGE ( 'NONE', *, *, #5993, .T. ) ;
#4581=AXIS2_PLACEMENT_3D ( 'NONE', #76, #10070, #682 ) ;
#4583=VECTOR ( 'NONE', #6018, 1000.000000000000000 ) ;
#4584=CARTESIAN_POINT ( 'NONE',  ( 9.875000000000023093, -0.001000000000001000089, 17.10400172474264835 ) ) ;
#4589=EDGE_CURVE ( 'NONE', #6120, #10105, #5313, .T. ) ;
#4591=ADVANCED_FACE ( 'NONE', ( #5416 ), #8001, .F. ) ;
#4594=ADVANCED_FACE ( 'NONE', ( #8774 ), #8729, .F. ) ;
#4599=DIRECTION ( 'NONE',  ( 0.000000000000000000, 0.000000000000000000, 1.000000000000000000 ) ) ;
#4601=ORIENTED_EDGE ( 'NONE', *, *, #7205, .T. ) ;
#4603=AXIS2_PLACEMENT_3D ( 'NONE', #2753, #6147, #5324 ) ;
#4609=CYLINDRICAL_SURFACE ( 'NONE', #1955, 2.999999999999997335 ) ;
#4616=VECTOR ( 'NONE', #3467, 1000.000000000000000 ) ;
#4619=CARTESIAN_POINT ( 'NONE',  ( -10.19839929293505776, 4.706249999044086252, -24.62111388750000174 ) ) ;
#4620=CARTESIAN_POINT ( 'NONE',  ( 10.35533905932738286, 3.812500000000000000, 24.99999999999999645 ) ) ;
#4621=VECTOR ( 'NONE', #522, 1000.000000000000000 ) ;
#4626=CARTESIAN_POINT ( 'NONE',  ( 3.957930336368489021E-15, 25.00000000000000000, 19.75000000000000000 ) ) ;
#4627=VERTEX_POINT ( 'NONE', #8669 ) ;
#4629=AXIS2_PLACEMENT_3D ( 'NONE', #9794, #7019, #215 ) ;
#4632=ORIENTED_EDGE ( 'NONE', *, *, #7486, .T. ) ;
#4636=DIRECTION ( 'NONE',  ( -0.000000000000000000, 1.000000000000000000, -0.000000000000000000 ) ) ;
#4638=ORIENTED_EDGE ( 'NONE', *, *, #520, .T. ) ;
#4642=EDGE_CURVE ( 'NONE', #10846, #5785, #10745, .T. ) ;
#4646=DIRECTION ( 'NONE',  ( 0.000000000000000000, 0.000000000000000000, 1.000000000000000000 ) ) ;
#4647=DIRECTION ( 'NONE',  ( 0.000000000000000000, 0.000000000000000000, 1.000000000000000000 ) ) ;
#4650=CIRCLE ( 'NONE', #5694, 25.00000000000000000 ) ;
#4652=VECTOR ( 'NONE', #4636, 1000.000000000000000 ) ;
#4654=CIRCLE ( 'NONE', #3200, 2.999999999999996447 ) ;
#4658=CARTESIAN_POINT ( 'NONE',  ( -10.19839929293505776, 2.706249999044084475, -24.62111388750000174 ) ) ;
#4659=VERTEX_POINT ( 'NONE', #3159 ) ;
#4661=LINE ( 'NONE', #9722, #6522 ) ;
#4663=LINE ( 'NONE', #2960, #2874 ) ;
#4668=AXIS2_PLACEMENT_3D ( 'NONE', #1042, #4415, #209 ) ;
#4670=ORIENTED_EDGE ( 'NONE', *, *, #7885, .F. ) ;
#4671=EDGE_LOOP ( 'NONE', ( #8837, #1106, #745, #8110 ) ) ;
#4675=CARTESIAN_POINT ( 'NONE',  ( 10.19839929293506486, 4.206249999044085364, 24.62111388749999819 ) ) ;
#4676=EDGE_LOOP ( 'NONE', ( #841, #5671, #5845, #6214 ) ) ;
#4678=CARTESIAN_POINT ( 'NONE',  ( -17.67766952966368876, 3.375000000000000000, -17.67766952966369232 ) ) ;
#4679=CARTESIAN_POINT ( 'NONE',  ( -4.592425496802574367E-15, 1.362499998088169129, 25.00000000000000000 ) ) ;
#4681=CARTESIAN_POINT ( 'NONE',  ( -4.592425496802574367E-15, 0.7500000000000000000, 25.00000000000000000 ) ) ;
#4689=DIRECTION ( 'NONE',  ( 0.000000000000000000, -0.000000000000000000, 1.000000000000000000 ) ) ;
#4690=CYLINDRICAL_SURFACE ( 'NONE', #6082, 2.999999999999997780 ) ;
#4697=DIRECTION ( 'NONE',  ( 0.000000000000000000, 0.000000000000000000, -1.000000000000000000 ) ) ;
#4699=DIRECTION ( 'NONE',  ( 0.000000000000000000, 1.000000000000000000, 0.000000000000000000 ) ) ;
#4701=DIRECTION ( 'NONE',  ( 1.000000000000000000, 0.000000000000000000, -1.069128445102650095E-14 ) ) ;
#4703=ORIENTED_EDGE ( 'NONE', *, *, #10240, .F. ) ;
#4705=DIRECTION ( 'NONE',  ( 0.000000000000000000, 0.000000000000000000, 1.000000000000000000 ) ) ;
#4706=CARTESIAN_POINT ( 'NONE',  ( 24.62111388750000174, 3.393749999044084475, 0.000000000000000000 ) ) ;
#4708=CARTESIAN_POINT ( 'NONE',  ( -12.13990010960501031, 25.00000000000000000, -10.47307621135320410 ) ) ;
#4709=EDGE_CURVE ( 'NONE', #4627, #4897, #4072, .T. ) ;
#4718=CARTESIAN_POINT ( 'NONE',  ( 17.40975659021752620, 1.268749999044084698, 17.40975659021753330 ) ) ;
#4719=ORIENTED_EDGE ( 'NONE', *, *, #2274, .T. ) ;
#4720=CARTESIAN_POINT ( 'NONE',  ( -10.35533905932739174, 3.687500000000000444, 24.99999999999999289 ) ) ;
#4721=EDGE_CURVE ( 'NONE', #5726, #8379, #6454, .T. ) ;
#4728=ORIENTED_EDGE ( 'NONE', *, *, #8877, .T. ) ;
#4731=CARTESIAN_POINT ( 'NONE',  ( -25.00000000000000000, 4.500000000000000888, -3.061616997868383043E-15 ) ) ;
#4734=VECTOR ( 'NONE', #10823, 1000.000000000000000 ) ;
#4736=DIRECTION ( 'NONE',  ( -0.000000000000000000, 1.000000000000000000, -0.000000000000000000 ) ) ;
#4742=VERTEX_POINT ( 'NONE', #3104 ) ;
#4744=VECTOR ( 'NONE', #5173, 1000.000000000000000 ) ;
#4745=DIRECTION ( 'NONE',  ( -0.8660254037844327124, 0.000000000000000000, 0.5000000000000103251 ) ) ;
#4749=CARTESIAN_POINT ( 'NONE',  ( 3.223142256880076948E-15, 28.00000000000000000, 15.75000000000000000 ) ) ;
#4754=CARTESIAN_POINT ( 'NONE',  ( 10.19839929293506486, 3.206249999044084031, 24.62111388749999819 ) ) ;
#4755=ORIENTED_EDGE ( 'NONE', *, *, #3823, .F. ) ;
#4756=CARTESIAN_POINT ( 'NONE',  ( 15.60400172474260927, 25.00000000000000000, -12.47307621135339062 ) ) ;
#4761=CARTESIAN_POINT ( 'NONE',  ( 1.530808498934191521E-15, 2.862499998088169573, -25.00000000000000000 ) ) ;
#4763=ORIENTED_EDGE ( 'NONE', *, *, #3333, .F. ) ;
#4768=CARTESIAN_POINT ( 'NONE',  ( 17.40975659021752975, 2.518749999044084475, -17.40975659021752975 ) ) ;
#4769=CARTESIAN_POINT ( 'NONE',  ( 17.67766952966369232, 3.125000000000000000, -17.67766952966369232 ) ) ;
#4772=CARTESIAN_POINT ( 'NONE',  ( -3.223142256880076948E-15, -0.001000000000001000089, -15.75000000000000000 ) ) ;
#4773=DIRECTION ( 'NONE',  ( -0.8660254037844328234, 0.000000000000000000, 0.5000000000000098810 ) ) ;
#4775=PLANE ( 'NONE',  #4230 ) ;
#4776=AXIS2_PLACEMENT_3D ( 'NONE', #545, #3279, #10038 ) ;
#4781=EDGE_CURVE ( 'NONE', #7939, #7899, #8372, .T. ) ;
#4782=ORIENTED_EDGE ( 'NONE', *, *, #10369, .T. ) ;
#4784=CIRCLE ( 'NONE', #201, 5.999999999999999112 ) ;
#4786=DIRECTION ( 'NONE',  ( 0.000000000000000000, 0.9230769230769232392, 0.3846153846153844702 ) ) ;
#4787=( LENGTH_UNIT ( ) NAMED_UNIT ( * ) SI_UNIT ( .MILLI., .METRE. ) );
#4789=DIRECTION ( 'NONE',  ( 1.000000000000000000, 0.000000000000000000, 0.000000000000000000 ) ) ;
#4790=DIRECTION ( 'NONE',  ( 0.000000000000000000, 1.000000000000000000, 0.000000000000000000 ) ) ;
#4793=VECTOR ( 'NONE', #4026, 1000.000000000000000 ) ;
#4795=ORIENTED_EDGE ( 'NONE', *, *, #5590, .F. ) ;
#4796=EDGE_CURVE ( 'NONE', #9663, #10596, #9366, .T. ) ;
#4798=VERTEX_POINT ( 'NONE', #5023 ) ;
#4801=DIRECTION ( 'NONE',  ( 0.000000000000000000, 0.000000000000000000, 1.000000000000000000 ) ) ;
#4802=AXIS2_PLACEMENT_3D ( 'NONE', #8465, #10801, #3373 ) ;
#4807=AXIS2_PLACEMENT_3D ( 'NONE', #1343, #8077, #511 ) ;
#4809=DIRECTION ( 'NONE',  ( -0.5000000000000073275, 0.000000000000000000, -0.8660254037844344888 ) ) ;
#4810=CARTESIAN_POINT ( 'NONE',  ( -24.62111388750000174, 2.831249999044084475, -10.19839929293506131 ) ) ;
#4811=EDGE_LOOP ( 'NONE', ( #7794, #5696, #1859, #7783, #6841 ) ) ;
#4816=CARTESIAN_POINT ( 'NONE',  ( -17.40975659021753330, 2.843749999044085097, 17.40975659021752975 ) ) ;
#4818=ADVANCED_FACE ( 'NONE', ( #88 ), #7596, .F. ) ;
#4826=CARTESIAN_POINT ( 'NONE',  ( 17.40975659021752975, 1.343749999044084653, -17.40975659021752975 ) ) ;
#4828=DIRECTION ( 'NONE',  ( 0.000000000000000000, 0.000000000000000000, -1.000000000000000000 ) ) ;
#4829=SHAPE_REPRESENTATION_RELATIONSHIP ( 'NONE' , 'NONE' ,  #5021, #715 ) ;
#4832=CARTESIAN_POINT ( 'NONE',  ( 24.99999999999999289, 1.549999998088169129, 10.35533905932739529 ) ) ;
#4838=VERTEX_POINT ( 'NONE', #4178 ) ;
#4842=VECTOR ( 'NONE', #1411, 1000.000000000000000 ) ;
#4846=CARTESIAN_POINT ( 'NONE',  ( 0.000000000000000000, 31.00000000000000000, 0.000000000000000000 ) ) ;
#4852=EDGE_CURVE ( 'NONE', #10741, #1857, #9409, .T. ) ;
#4859=( BOUNDED_CURVE ( )  B_SPLINE_CURVE ( 2, ( #8693, #1139, #126, #4518, #10235 ),
 .UNSPECIFIED., .F., .F. ) 
 B_SPLINE_CURVE_WITH_KNOTS ( ( 3, 2, 3 ),
 ( 0.000000000000000000, 0.02500000000000000486, 0.05000000000000000971 ),
 .UNSPECIFIED. ) 
 CURVE ( )  GEOMETRIC_REPRESENTATION_ITEM ( )  RATIONAL_B_SPLINE_CURVE ( ( 1.000000000000000000, 0.9238795325112867385, 1.000000000000000000, 0.9238795325112867385, 1.000000000000000000 ) ) 
 REPRESENTATION_ITEM ( '' )  );
#4860=CARTESIAN_POINT ( 'NONE',  ( 10.35533905932734733, 4.187500000000000888, -25.00000000000004263 ) ) ;
#4861=CARTESIAN_POINT ( 'NONE',  ( 0.000000000000000000, 27.99999999999999645, -25.00000000000000000 ) ) ;
#4864=DIRECTION ( 'NONE',  ( 0.000000000000000000, 1.000000000000000000, 0.000000000000000000 ) ) ;
#4866=CARTESIAN_POINT ( 'NONE',  ( -10.19839929293507375, 3.081249999044084920, 24.62111388749999108 ) ) ;
#4872=CARTESIAN_POINT ( 'NONE',  ( 17.40975659021752975, 0.3437499990440845421, -17.40975659021752975 ) ) ;
#4877=CARTESIAN_POINT ( 'NONE',  ( -10.19839929293505776, 0.5312499990440845421, -24.62111388750000174 ) ) ;
#4882=DIRECTION ( 'NONE',  ( 0.000000000000000000, 0.000000000000000000, 1.000000000000000000 ) ) ;
#4883=LINE ( 'NONE', #9071, #2832 ) ;
#4884=EDGE_LOOP ( 'NONE', ( #6331, #9808, #7708, #4535 ) ) ;
#4886=CARTESIAN_POINT ( 'NONE',  ( 24.62111388750000174, 2.218749999044084653, 0.000000000000000000 ) ) ;
#4895=ORIENTED_EDGE ( 'NONE', *, *, #1336, .T. ) ;
#4897=VERTEX_POINT ( 'NONE', #8536 ) ;
#4909=ADVANCED_FACE ( 'NONE', ( #2938 ), #9061, .F. ) ;
#4913=LINE ( 'NONE', #3456, #5162 ) ;
#4918=ORIENTED_EDGE ( 'NONE', *, *, #7546, .F. ) ;
#4922=CARTESIAN_POINT ( 'NONE',  ( -17.40975659021752975, 1.593749999044084431, -17.40975659021752975 ) ) ;
#4929=CARTESIAN_POINT ( 'NONE',  ( 17.40975659021752975, 3.343749999044085097, -17.40975659021752975 ) ) ;
#4930=EDGE_LOOP ( 'NONE', ( #6773, #9877, #513, #8584 ) ) ;
#4933=FACE_OUTER_BOUND ( 'NONE', #794, .T. ) ;
#4943=CARTESIAN_POINT ( 'NONE',  ( 10.19839929293506486, 3.206249999044084031, 24.62111388749999819 ) ) ;
#4946=CIRCLE ( 'NONE', #3701, 2.999999999999999112 ) ;
#4947=ADVANCED_FACE ( 'NONE', ( #2836 ), #1919, .F. ) ;
#4958=EDGE_LOOP ( 'NONE', ( #7001, #10808, #5594, #4530 ) ) ;
#4959=CARTESIAN_POINT ( 'NONE',  ( 0.000000000000000000, 85.00000000000000000, 0.000000000000000000 ) ) ;
#4962=CIRCLE ( 'NONE', #1966, 2.999999999999998668 ) ;
#4964=CARTESIAN_POINT ( 'NONE',  ( 1.530808498934191521E-15, 4.250000000000000000, -25.00000000000000000 ) ) ;
#4967=ORIENTED_EDGE ( 'NONE', *, *, #3148, .F. ) ;
#4970=VECTOR ( 'NONE', #6167, 1000.000000000000000 ) ;
#4971=CARTESIAN_POINT ( 'NONE',  ( -15.74999999999997158, 25.00000000000000000, 3.000000000000162981 ) ) ;
#4977=CARTESIAN_POINT ( 'NONE',  ( -24.62111388750000174, 0.6562499990440845421, -10.19839929293506131 ) ) ;
#4978=ADVANCED_FACE ( 'NONE', ( #1980 ), #6123, .F. ) ;
#4982=EDGE_CURVE ( 'NONE', #634, #7970, #6340, .T. ) ;
#4985=CARTESIAN_POINT ( 'NONE',  ( 17.40975659021752975, 2.343749999044085097, -17.40975659021752975 ) ) ;
#4986=DIRECTION ( 'NONE',  ( 0.000000000000000000, 1.000000000000000000, -0.000000000000000000 ) ) ;
#4987=EDGE_LOOP ( 'NONE', ( #2565, #5464, #8523, #7870 ) ) ;
#4990=LINE ( 'NONE', #6589, #5966 ) ;
#4993=DIRECTION ( 'NONE',  ( 0.8660254037844451469, 0.000000000000000000, 0.4999999999999887312 ) ) ;
#4997=ORIENTED_EDGE ( 'NONE', *, *, #4473, .F. ) ;
#4999=ORIENTED_EDGE ( 'NONE', *, *, #3833, .T. ) ;
#5001=ORIENTED_EDGE ( 'NONE', *, *, #9891, .T. ) ;
#5002=CARTESIAN_POINT ( 'NONE',  ( -10.35533905932739174, 5.299999998088169129, 24.99999999999999289 ) ) ;
#5003=AXIS2_PLACEMENT_3D ( 'NONE', #8916, #3044, #7209 ) ;
#5005=CARTESIAN_POINT ( 'NONE',  ( -7.276923788646446845, 25.00000000000000000, 18.60400172474275848 ) ) ;
#5009=FACE_BOUND ( 'NONE', #10247, .T. ) ;
#5013=CARTESIAN_POINT ( 'NONE',  ( 7.276923788646707969, 28.00000000000000000, 18.60400172474265190 ) ) ;
#5016=AXIS2_PLACEMENT_3D ( 'NONE', #4348, #814, #2500 ) ;
#5017=VERTEX_POINT ( 'NONE', #6237 ) ;
#5021=SHAPE_REPRESENTATION ( 'Upper Stainless Steel Body Shell', ( #7040 ), #6327 ) ;
#5023=CARTESIAN_POINT ( 'NONE',  ( 15.75000000000001421, 28.00000000000000000, 2.999999999999942268 ) ) ;
#5024=CARTESIAN_POINT ( 'NONE',  ( 15.13990010960492505, 25.00000000000000000, 5.276923788646651126 ) ) ;
#5025=CARTESIAN_POINT ( 'NONE',  ( 0.000000000000000000, 20.00000000000000355, 0.000000000000000000 ) ) ;
#5029=CARTESIAN_POINT ( 'NONE',  ( -17.67766952966369232, 4.237499998088169129, 17.67766952966368876 ) ) ;
#5034=CARTESIAN_POINT ( 'NONE',  ( 17.10400172474269098, -0.001000000000001000089, 12.87499999999995381 ) ) ;
#5036=CARTESIAN_POINT ( 'NONE',  ( 24.62111388750000174, 3.218749999044084653, 0.000000000000000000 ) ) ;
#5041=CARTESIAN_POINT ( 'NONE',  ( 17.40975659021752975, 0.3437499990440845421, -17.40975659021752975 ) ) ;
#5044=CARTESIAN_POINT ( 'NONE',  ( -3.223142256880076948E-15, 28.00000000000000000, -15.75000000000000000 ) ) ;
#5046=CARTESIAN_POINT ( 'NONE',  ( -18.60400172474257730, 28.00000000000000000, 7.276923788646904256 ) ) ;
#5047=CARTESIAN_POINT ( 'NONE',  ( 3.061616997868383043E-15, 8.000000000000003553, 25.00000000000000000 ) ) ;
#5052=ADVANCED_FACE ( 'NONE', ( #5354 ), #5499, .F. ) ;
#5054=VERTEX_POINT ( 'NONE', #1098 ) ;
#5055=VERTEX_POINT ( 'NONE', #3623 ) ;
#5056=EDGE_CURVE ( 'NONE', #2069, #6402, #2780, .T. ) ;
#5057=CARTESIAN_POINT ( 'NONE',  ( 13.63990010960487353, 25.00000000000000000, -7.875000000000067502 ) ) ;
#5059=CARTESIAN_POINT ( 'NONE',  ( 10.19839929293506486, 2.206249999044084920, 24.62111388749999819 ) ) ;
#5060=CARTESIAN_POINT ( 'NONE',  ( 24.62111388749999463, 1.156249999044084431, 10.19839929293507730 ) ) ;
#5067=VERTEX_POINT ( 'NONE', #9797 ) ;
#5068=VERTEX_POINT ( 'NONE', #3957 ) ;
#5076=CARTESIAN_POINT ( 'NONE',  ( 24.81055694375000087, 0.5031249985661269131, 0.000000000000000000 ) ) ;
#5077=CARTESIAN_POINT ( 'NONE',  ( 3.957930336368489021E-15, 25.00000000000000000, 19.75000000000000000 ) ) ;
#5081=DIRECTION ( 'NONE',  ( 0.8660254037844399289, -0.000000000000000000, 0.4999999999999977796 ) ) ;
#5082=ORIENTED_EDGE ( 'NONE', *, *, #1623, .F. ) ;
#5083=FACE_OUTER_BOUND ( 'NONE', #1770, .T. ) ;
#5084=CARTESIAN_POINT ( 'NONE',  ( 0.000000000000000000, 28.00000000000000000, -5.999999999999999112 ) ) ;
#5087=VERTEX_POINT ( 'NONE', #1353 ) ;
#5088=VECTOR ( 'NONE', #9126, 1000.000000000000000 ) ;
#5089=CARTESIAN_POINT ( 'NONE',  ( -15.60400172474251868, 25.00000000000000000, 12.47307621135349720 ) ) ;
#5091=PLANE ( 'NONE',  #2177 ) ;
#5093=CARTESIAN_POINT ( 'NONE',  ( -4.592425496802574367E-15, 3.750000000000000000, 25.00000000000000000 ) ) ;
#5100=ORIENTED_EDGE ( 'NONE', *, *, #3392, .T. ) ;
#5105=ADVANCED_FACE ( 'NONE', ( #2992 ), #4690, .F. ) ;
#5106=CARTESIAN_POINT ( 'NONE',  ( -24.62111388750000174, 0.8937499990440845865, -3.015216831376932151E-15 ) ) ;
#5107=CARTESIAN_POINT ( 'NONE',  ( 17.67766952966368521, 0.8750000000000000000, 17.67766952966369232 ) ) ;
#5114=EDGE_CURVE ( 'NONE', #6661, #5087, #9078, .T. ) ;
#5116=ORIENTED_EDGE ( 'NONE', *, *, #8153, .T. ) ;
#5122=DIRECTION ( 'NONE',  ( -0.000000000000000000, 1.000000000000000000, -0.000000000000000000 ) ) ;
#5125=CARTESIAN_POINT ( 'NONE',  ( 12.47307621135322186, 25.00000000000000000, -15.60400172474273717 ) ) ;
#5133=ORIENTED_EDGE ( 'NONE', *, *, #3561, .T. ) ;
#5134=EDGE_LOOP ( 'NONE', ( #4162, #8367, #10754, #3993 ) ) ;
#5138=CIRCLE ( 'NONE', #696, 28.00000000000000000 ) ;
#5139=DIRECTION ( 'NONE',  ( 0.000000000000000000, 0.000000000000000000, 1.000000000000000000 ) ) ;
#5141=PRODUCT_CONTEXT ( 'NONE', #3263, 'mechanical' ) ;
#5144=EDGE_CURVE ( 'NONE', #5055, #8118, #1311, .T. ) ;
#5145=FACE_BOUND ( 'NONE', #5278, .T. ) ;
#5146=DIRECTION ( 'NONE',  ( 0.000000000000000000, 1.000000000000000000, -0.000000000000000000 ) ) ;
#5148=( BOUNDED_CURVE ( )  B_SPLINE_CURVE ( 2, ( #1363, #3270, #642, #7431, #6615, #1573, #10814, #4860, #4964 ),
 .UNSPECIFIED., .F., .F. ) 
 B_SPLINE_CURVE_WITH_KNOTS ( ( 3, 2, 2, 2, 3 ),
 ( 0.7500000000000000000, 0.7750000000000000222, 0.8000000000000000444, 0.8250000000000000666, 0.8500000000000000888 ),
 .UNSPECIFIED. ) 
 CURVE ( )  GEOMETRIC_REPRESENTATION_ITEM ( )  RATIONAL_B_SPLINE_CURVE ( ( 1.000000000000000000, 0.9238795325112867385, 1.000000000000000000, 0.9238795325112867385, 1.000000000000000000, 0.9238795325112867385, 1.000000000000000000, 0.9238795325112864054, 1.000000000000000444 ) ) 
 REPRESENTATION_ITEM ( '' )  );
#5151=CARTESIAN_POINT ( 'NONE',  ( 10.35533905932738286, 2.812500000000000000, 24.99999999999999645 ) ) ;
#5154=CARTESIAN_POINT ( 'NONE',  ( -4.592425496802574367E-15, 1.362499998088169129, 25.00000000000000000 ) ) ;
#5161=ORIENTED_EDGE ( 'NONE', *, *, #1135, .F. ) ;
#5162=VECTOR ( 'NONE', #5081, 1000.000000000000114 ) ;
#5163=ORIENTED_EDGE ( 'NONE', *, *, #10771, .F. ) ;
#5165=ORIENTED_EDGE ( 'NONE', *, *, #3849, .T. ) ;
#5166=CARTESIAN_POINT ( 'NONE',  ( 0.000000000000000000, 85.00000000000000000, 0.000000000000000000 ) ) ;
#5169=CARTESIAN_POINT ( 'NONE',  ( 24.62111388750000174, 0.4562499990440845865, -10.19839929293505776 ) ) ;
#5170=CARTESIAN_POINT ( 'NONE',  ( -10.19839929293505776, 2.706249999044084475, -24.62111388750000174 ) ) ;
#5171=CARTESIAN_POINT ( 'NONE',  ( 10.35533905932737930, 1.187500000000000444, -25.00000000000000000 ) ) ;
#5172=FILL_AREA_STYLE ('',( #6823 ) ) ;
#5173=DIRECTION ( 'NONE',  ( -0.000000000000000000, 1.000000000000000000, -0.000000000000000000 ) ) ;
#5174=CIRCLE ( 'NONE', #3933, 7.500000000000000888 ) ;
#5176=FACE_OUTER_BOUND ( 'NONE', #6926, .T. ) ;
#5180=ORIENTED_EDGE ( 'NONE', *, *, #3616, .F. ) ;
#5181=CIRCLE ( 'NONE', #3752, 25.00000000000000000 ) ;
#5191=DIRECTION ( 'NONE',  ( -1.000000000000000000, 0.000000000000000000, -0.000000000000000000 ) ) ;
#5194=DIRECTION ( 'NONE',  ( 0.000000000000000000, 0.000000000000000000, 1.000000000000000000 ) ) ;
#5196=CARTESIAN_POINT ( 'NONE',  ( 7.347880794884118750E-16, 25.00000000000000000, 5.999999999999999112 ) ) ;
#5200=EDGE_CURVE ( 'NONE', #7304, #2289, #3150, .T. ) ;
#5202=ORIENTED_EDGE ( 'NONE', *, *, #9998, .T. ) ;
#5206=DIRECTION ( 'NONE',  ( -0.000000000000000000, -1.000000000000000000, -0.000000000000000000 ) ) ;
#5209=LINE ( 'NONE', #5034, #1305 ) ;
#5210=CARTESIAN_POINT ( 'NONE',  ( -17.67766952966368876, 4.987499998088170017, -17.67766952966369232 ) ) ;
#5211=EDGE_CURVE ( 'NONE', #5055, #9481, #6392, .T. ) ;
#5214=CARTESIAN_POINT ( 'NONE',  ( 0.000000000000000000, 28.00000000000000000, -5.999999999999999112 ) ) ;
#5215=CARTESIAN_POINT ( 'NONE',  ( 24.99999999999999289, 2.937500000000000000, 10.35533905932739529 ) ) ;
#5218=CARTESIAN_POINT ( 'NONE',  ( -25.00000000000000000, 3.500000000000000000, -3.061616997868383043E-15 ) ) ;
#5223=CYLINDRICAL_SURFACE ( 'NONE', #1809, 2.999999999999997335 ) ;
#5225=( BOUNDED_CURVE ( )  B_SPLINE_CURVE ( 2, ( #9222, #3533, #6699, #6928, #10286, #10055, #2968, #2702, #6099 ),
 .UNSPECIFIED., .F., .F. ) 
 B_SPLINE_CURVE_WITH_KNOTS ( ( 3, 2, 2, 2, 3 ),
 ( 0.1499999999999999944, 0.1749999999999999889, 0.2000000000000000111, 0.2249999999999999778, 0.2499999999999999722 ),
 .UNSPECIFIED. ) 
 CURVE ( )  GEOMETRIC_REPRESENTATION_ITEM ( )  RATIONAL_B_SPLINE_CURVE ( ( 1.000000000000000000, 0.9238795325112867385, 1.000000000000000000, 0.9238795325112867385, 1.000000000000000000, 0.9238795325112867385, 1.000000000000000000, 0.9238795325112868495, 0.9999999999999998890 ) ) 
 REPRESENTATION_ITEM ( '' )  );
#5228=CYLINDRICAL_SURFACE ( 'NONE', #6338, 7.500000000000000888 ) ;
#5230=CARTESIAN_POINT ( 'NONE',  ( -2.999999999999999112, 25.00000000000000000, -19.75000000000000000 ) ) ;
#5231=CARTESIAN_POINT ( 'NONE',  ( 25.00000000000000000, 4.612499998088169129, 0.000000000000000000 ) ) ;
#5232=CARTESIAN_POINT ( 'NONE',  ( 24.62111388749999463, 5.156249999044083765, 10.19839929293507730 ) ) ;
#5233=DIRECTION ( 'NONE',  ( 0.000000000000000000, 0.000000000000000000, 1.000000000000000000 ) ) ;
#5237=DIRECTION ( 'NONE',  ( 0.000000000000000000, 0.000000000000000000, 1.000000000000000000 ) ) ;
#5240=VERTEX_POINT ( 'NONE', #9960 ) ;
#5241=EDGE_LOOP ( 'NONE', ( #3363, #8183, #9243, #8626 ) ) ;
#5242=VERTEX_POINT ( 'NONE', #7744 ) ;
#5243=CARTESIAN_POINT ( 'NONE',  ( 15.60400172474269453, 25.00000000000000000, 12.47307621135327693 ) ) ;
#5244=CARTESIAN_POINT ( 'NONE',  ( 19.75000000000000000, 28.00000000000000000, -7.291468677852036884E-14 ) ) ;
#5252=CARTESIAN_POINT ( 'NONE',  ( -10.19839929293507552, 5.081249999044084475, 24.62111388749999463 ) ) ;
#5253=EDGE_LOOP ( 'NONE', ( #2522, #8627, #10665, #1 ) ) ;
#5265=CARTESIAN_POINT ( 'NONE',  ( 17.40975659021752620, 5.093749999044084653, 17.40975659021753330 ) ) ;
#5266=CARTESIAN_POINT ( 'NONE',  ( -10.19839929293507375, 1.081249999044084475, 24.62111388749999108 ) ) ;
#5268=ADVANCED_FACE ( 'NONE', ( #3653 ), #1950, .F. ) ;
#5269=CARTESIAN_POINT ( 'NONE',  ( -25.00000000000000000, 3.437500000000000000, -10.35533905932738108 ) ) ;
#5272=CARTESIAN_POINT ( 'NONE',  ( 0.000000000000000000, 28.00000000000000000, 0.000000000000000000 ) ) ;
#5276=ORIENTED_EDGE ( 'NONE', *, *, #1732, .F. ) ;
#5278=EDGE_LOOP ( 'NONE', ( #2752, #3631 ) ) ;
#5282=CARTESIAN_POINT ( 'NONE',  ( 0.000000000000000000, 0.000000000000000000, -25.00000000000000000 ) ) ;
#5283=CARTESIAN_POINT ( 'NONE',  ( 17.67766952966369232, 3.737499998088169573, -17.67766952966369232 ) ) ;
#5284=CARTESIAN_POINT ( 'NONE',  ( 17.40975659021752975, 4.343749999044084653, -17.40975659021752975 ) ) ;
#5287=LINE ( 'NONE', #4460, #8611 ) ;
#5288=DIRECTION ( 'NONE',  ( -0.000000000000000000, 1.000000000000000000, -0.000000000000000000 ) ) ;
#5291=VECTOR ( 'NONE', #6045, 1000.000000000000000 ) ;
#5295=VERTEX_POINT ( 'NONE', #2438 ) ;
#5300=DIRECTION ( 'NONE',  ( -0.000000000000000000, -1.000000000000000000, -0.000000000000000000 ) ) ;
#5302=ADVANCED_FACE ( 'NONE', ( #4443, #6864, #741, #7865, #10288, #9517, #6653, #8564, #5009, #1012, #2703, #802, #10222, #3255 ), #2640, .T. ) ;
#5303=DIRECTION ( 'NONE',  ( -0.8660254037844327124, 0.000000000000000000, 0.5000000000000103251 ) ) ;
#5304=DIRECTION ( 'NONE',  ( 0.000000000000000000, 0.000000000000000000, 1.000000000000000000 ) ) ;
#5305=CARTESIAN_POINT ( 'NONE',  ( 10.19839929293506486, 4.206249999044084475, 24.62111388749999819 ) ) ;
#5306=ORIENTED_EDGE ( 'NONE', *, *, #2274, .F. ) ;
#5307=ORIENTED_EDGE ( 'NONE', *, *, #4385, .F. ) ;
#5313=CIRCLE ( 'NONE', #2351, 2.999999999999999112 ) ;
#5315=DIRECTION ( 'NONE',  ( 0.8660254037844327124, 0.000000000000000000, -0.5000000000000103251 ) ) ;
#5316=CARTESIAN_POINT ( 'NONE',  ( 17.10400172474269098, 28.00000000000000000, 12.87499999999995559 ) ) ;
#5317=ADVANCED_FACE ( 'NONE', ( #6100 ), #4511, .F. ) ;
#5320=CARTESIAN_POINT ( 'NONE',  ( 19.74999999999998934, 28.00000000000000000, -3.000000000000067946 ) ) ;
#5321=CARTESIAN_POINT ( 'NONE',  ( 24.62111388749999463, 5.156249999044083765, 10.19839929293507730 ) ) ;
#5322=CARTESIAN_POINT ( 'NONE',  ( 10.19839929293505953, 0.5812499990440844755, -24.62111388750000174 ) ) ;
#5324=DIRECTION ( 'NONE',  ( 0.8660254037844327124, 0.000000000000000000, -0.5000000000000103251 ) ) ;
#5326=CARTESIAN_POINT ( 'NONE',  ( -25.00000000000000000, 2.500000000000000000, -3.061616997868383043E-15 ) ) ;
#5327=DIRECTION ( 'NONE',  ( -1.000000000000000000, 0.000000000000000000, 1.069128445102650095E-14 ) ) ;
#5330=CIRCLE ( 'NONE', #3905, 15.00000000000000178 ) ;
#5332=ORIENTED_EDGE ( 'NONE', *, *, #6602, .T. ) ;
#5336=CARTESIAN_POINT ( 'NONE',  ( -25.00000000000000000, 3.112499998088169129, -3.061616997868383043E-15 ) ) ;
#5337=CARTESIAN_POINT ( 'NONE',  ( 17.67766952966369232, 0.1249999999999999722, -17.67766952966369232 ) ) ;
#5338=CARTESIAN_POINT ( 'NONE',  ( -2.999999999999999112, -0.001000000000001000089, -19.75000000000000000 ) ) ;
#5348=ORIENTED_EDGE ( 'NONE', *, *, #1157, .F. ) ;
#5349=CARTESIAN_POINT ( 'NONE',  ( 0.000000000000000000, 85.00000000000000000, -25.00000000000000000 ) ) ;
#5350=EDGE_CURVE ( 'NONE', #3918, #9337, #5698, .T. ) ;
#5352=PLANE ( 'NONE',  #8509 ) ;
#5354=FACE_OUTER_BOUND ( 'NONE', #3362, .T. ) ;
#5355=CIRCLE ( 'NONE', #565, 28.00000000000000000 ) ;
#5356=DIRECTION ( 'NONE',  ( 0.000000000000000000, 1.000000000000000000, -0.000000000000000000 ) ) ;
#5358=CARTESIAN_POINT ( 'NONE',  ( 0.000000000000000000, 31.00000000000000000, 0.000000000000000000 ) ) ;
#5359=LINE ( 'NONE', #8482, #8117 ) ;
#5361=CARTESIAN_POINT ( 'NONE',  ( 24.62111388750000174, 5.393749999044085364, 0.000000000000000000 ) ) ;
#5363=AXIS2_PLACEMENT_3D ( 'NONE', #6150, #4324, #5821 ) ;
#5364=EDGE_LOOP ( 'NONE', ( #7918, #4632, #2301, #5375 ) ) ;
#5366=CARTESIAN_POINT ( 'NONE',  ( 0.000000000000000000, 85.00000000000000000, 0.000000000000000000 ) ) ;
#5371=AXIS2_PLACEMENT_3D ( 'NONE', #6503, #8312, #4134 ) ;
#5375=ORIENTED_EDGE ( 'NONE', *, *, #5200, .F. ) ;
#5377=VERTEX_POINT ( 'NONE', #5851 ) ;
#5380=CARTESIAN_POINT ( 'NONE',  ( -25.00000000000001066, 0.5625000000000002220, 10.35533905932737397 ) ) ;
#5381=CARTESIAN_POINT ( 'NONE',  ( -24.62111388750000884, 0.9562499990440846975, 10.19839929293505421 ) ) ;
#5384=DIRECTION ( 'NONE',  ( 0.000000000000000000, 1.000000000000000000, -0.000000000000000000 ) ) ;
#5386=EDGE_CURVE ( 'NONE', #120, #7041, #8383, .T. ) ;
#5387=DIRECTION ( 'NONE',  ( 0.000000000000000000, 0.000000000000000000, 1.000000000000000000 ) ) ;
#5390=LINE ( 'NONE', #5482, #4074 ) ;
#5392=CARTESIAN_POINT ( 'NONE',  ( 24.62111388749999463, 4.331249999044085364, 10.19839929293507730 ) ) ;
#5393=CARTESIAN_POINT ( 'NONE',  ( 1.530808498934191521E-15, 3.862499998088169573, -25.00000000000000000 ) ) ;
#5394=CARTESIAN_POINT ( 'NONE',  ( 25.00000000000000000, 2.062500000000000000, -10.35533905932737753 ) ) ;
#5397=CARTESIAN_POINT ( 'NONE',  ( 2.999999999999996447, -0.001000000000001000089, -19.75000000000000000 ) ) ;
#5398=DIRECTION ( 'NONE',  ( 0.000000000000000000, 0.000000000000000000, 1.000000000000000000 ) ) ;
#5399=CARTESIAN_POINT ( 'NONE',  ( 0.000000000000000000, 8.000000000000003553, -25.00000000000000000 ) ) ;
#5406=CARTESIAN_POINT ( 'NONE',  ( -18.60400172474273361, 25.00000000000000000, -7.276923788646511682 ) ) ;
#5413=EDGE_CURVE ( 'NONE', #6661, #5017, #3758, .T. ) ;
#5414=ORIENTED_EDGE ( 'NONE', *, *, #10369, .F. ) ;
#5416=FACE_OUTER_BOUND ( 'NONE', #10473, .T. ) ;
#5423=CARTESIAN_POINT ( 'NONE',  ( 17.67766952966369232, 3.125000000000000000, -17.67766952966369232 ) ) ;
#5426=FACE_OUTER_BOUND ( 'NONE', #8844, .T. ) ;
#5427=LINE ( 'NONE', #6148, #239 ) ;
#5429=CARTESIAN_POINT ( 'NONE',  ( 1.530808498934191521E-15, 2.250000000000000444, -25.00000000000000000 ) ) ;
#5434=VECTOR ( 'NONE', #7006, 1000.000000000000000 ) ;
#5435=CARTESIAN_POINT ( 'NONE',  ( 17.40975659021752620, 3.268749999044084475, 17.40975659021753330 ) ) ;
#5437=CARTESIAN_POINT ( 'NONE',  ( -25.00000000000000000, 2.500000000000000000, -3.061616997868383043E-15 ) ) ;
#5438=CARTESIAN_POINT ( 'NONE',  ( -13.63990010960498367, 28.00000000000000000, -7.874999999999870326 ) ) ;
#5443=VERTEX_POINT ( 'NONE', #1489 ) ;
#5450=DIRECTION ( 'NONE',  ( -0.000000000000000000, 1.000000000000000000, -0.000000000000000000 ) ) ;
#5453=DIRECTION ( 'NONE',  ( 0.8660254037844362651, 0.000000000000000000, -0.5000000000000041078 ) ) ;
#5455=EDGE_CURVE ( 'NONE', #3821, #1673, #6468, .T. ) ;
#5458=PLANE ( 'NONE',  #9865 ) ;
#5460=CYLINDRICAL_SURFACE ( 'NONE', #8179, 25.00000000000000000 ) ;
#5461=FACE_OUTER_BOUND ( 'NONE', #4987, .T. ) ;
#5462=CARTESIAN_POINT ( 'NONE',  ( 2.999999999999999112, 25.00000000000000000, 19.75000000000000000 ) ) ;
#5464=ORIENTED_EDGE ( 'NONE', *, *, #1331, .T. ) ;
#5468=CARTESIAN_POINT ( 'NONE',  ( -10.35533905932738108, 0.6875000000000002220, 24.99999999999999645 ) ) ;
#5470=CARTESIAN_POINT ( 'NONE',  ( 24.62111388750000174, 1.456249999044084920, -10.19839929293505776 ) ) ;
#5472=ORIENTED_EDGE ( 'NONE', *, *, #10924, .F. ) ;
#5481=VERTEX_POINT ( 'NONE', #103 ) ;
#5482=CARTESIAN_POINT ( 'NONE',  ( 0.000000000000000000, 85.00000000000000000, -25.00000000000000000 ) ) ;
#5484=CARTESIAN_POINT ( 'NONE',  ( 1.507608415688466075E-15, 1.643749999044084475, -24.62111388750000174 ) ) ;
#5485=ORIENTED_EDGE ( 'NONE', *, *, #3634, .F. ) ;
#5491=CARTESIAN_POINT ( 'NONE',  ( 25.00000000000000000, 0.6124999980881691286, 0.000000000000000000 ) ) ;
#5493=DIRECTION ( 'NONE',  ( 0.5000000000000012212, 0.000000000000000000, 0.8660254037844380415 ) ) ;
#5497=CIRCLE ( 'NONE', #2843, 2.999999999999997780 ) ;
#5499=CYLINDRICAL_SURFACE ( 'NONE', #2187, 25.00000000000000000 ) ;
#5504=CIRCLE ( 'NONE', #5682, 2.999999999999997335 ) ;
#5507=VECTOR ( 'NONE', #1121, 1000.000000000000000 ) ;
#5509=ORIENTED_EDGE ( 'NONE', *, *, #3895, .T. ) ;
#5511=LINE ( 'NONE', #7023, #8285 ) ;
#5516=ADVANCED_FACE ( 'NONE', ( #6850, #5145 ), #4312, .T. ) ;
#5517=VECTOR ( 'NONE', #5315, 1000.000000000000000 ) ;
#5522=AXIS2_PLACEMENT_3D ( 'NONE', #5949, #4296, #7659 ) ;
#5526=CARTESIAN_POINT ( 'NONE',  ( -4.522825247065398226E-15, 2.143749999044084920, 24.62111388750000174 ) ) ;
#5527=EDGE_LOOP ( 'NONE', ( #2095, #8234, #3278, #1284 ) ) ;
#5532=AXIS2_PLACEMENT_3D ( 'NONE', #8940, #9872, #9818 ) ;
#5535=ORIENTED_EDGE ( 'NONE', *, *, #2071, .T. ) ;
#5536=AXIS2_PLACEMENT_3D ( 'NONE', #5358, #1100, #10422 ) ;
#5542=LINE ( 'NONE', #790, #10250 ) ;
#5544=CARTESIAN_POINT ( 'NONE',  ( -17.40975659021752975, 2.768749999044084475, -17.40975659021752975 ) ) ;
#5545=ORIENTED_EDGE ( 'NONE', *, *, #2914, .F. ) ;
#5546=VECTOR ( 'NONE', #4736, 1000.000000000000000 ) ;
#5547=CARTESIAN_POINT ( 'NONE',  ( 10.35533905932737930, 3.187500000000000000, -25.00000000000000000 ) ) ;
#5549=CARTESIAN_POINT ( 'NONE',  ( 1.530808498934191521E-15, 1.862499998088169129, -25.00000000000000000 ) ) ;
#5550=DIRECTION ( 'NONE',  ( -0.000000000000000000, 1.000000000000000000, -0.000000000000000000 ) ) ;
#5556=ORIENTED_EDGE ( 'NONE', *, *, #7042, .T. ) ;
#5560=CARTESIAN_POINT ( 'NONE',  ( 0.000000000000000000, 31.00000000000000000, -10.50000000000000000 ) ) ;
#5563=CARTESIAN_POINT ( 'NONE',  ( -2.999999999999999112, 28.00000000000000000, -19.75000000000000000 ) ) ;
#5570=CARTESIAN_POINT ( 'NONE',  ( 10.35533905932738286, 4.424999998088169129, 24.99999999999999645 ) ) ;
#5575=EDGE_CURVE ( 'NONE', #5443, #4321, #3382, .T. ) ;
#5576=EDGE_CURVE ( 'NONE', #1857, #5785, #3585, .T. ) ;
#5579=CARTESIAN_POINT ( 'NONE',  ( 1.507608415688466075E-15, 3.643749999044084920, -24.62111388750000174 ) ) ;
#5580=ORIENTED_EDGE ( 'NONE', *, *, #9560, .F. ) ;
#5581=FACE_OUTER_BOUND ( 'NONE', #1033, .T. ) ;
#5585=DIRECTION ( 'NONE',  ( -0.000000000000000000, 1.000000000000000000, -0.000000000000000000 ) ) ;
#5586=EDGE_CURVE ( 'NONE', #416, #9664, #8671, .T. ) ;
#5590=EDGE_CURVE ( 'NONE', #5068, #10398, #2502, .T. ) ;
#5593=CARTESIAN_POINT ( 'NONE',  ( -10.19839929293507552, 2.081249999044084475, 24.62111388749999463 ) ) ;
#5594=ORIENTED_EDGE ( 'NONE', *, *, #3895, .F. ) ;
#5595=CARTESIAN_POINT ( 'NONE',  ( -25.00000000000001421, 1.562500000000000000, 10.35533905932737397 ) ) ;
#5596=PLANE ( 'NONE',  #2591 ) ;
#5599=CARTESIAN_POINT ( 'NONE',  ( 17.67766952966368521, 3.487499998088169129, 17.67766952966369232 ) ) ;
#5600=EDGE_CURVE ( 'NONE', #7830, #10741, #9758, .T. ) ;
#5603=ORIENTED_EDGE ( 'NONE', *, *, #1525, .T. ) ;
#5608=CARTESIAN_POINT ( 'NONE',  ( -17.67766952966369232, 4.625000000000000000, 17.67766952966368876 ) ) ;
#5609=COLOUR_RGB ( '', 0.09019608, 0.27058824, 0.51372549) ;
#5610=CARTESIAN_POINT ( 'NONE',  ( -9.874999999999777955, -0.001000000000001000089, 20.10400172474279401 ) ) ;
#5611=DIRECTION ( 'NONE',  ( 0.000000000000000000, 1.000000000000000000, 0.000000000000000000 ) ) ;
#5612=AXIS2_PLACEMENT_3D ( 'NONE', #7710, #2774, #4409 ) ;
#5614=DIRECTION ( 'NONE',  ( -0.000000000000000000, 1.000000000000000000, -0.000000000000000000 ) ) ;
#5615=ORIENTED_EDGE ( 'NONE', *, *, #4302, .F. ) ;
#5617=CIRCLE ( 'NONE', #4581, 2.999999999999998224 ) ;
#5618=ORIENTED_EDGE ( 'NONE', *, *, #6894, .T. ) ;
#5621=DIRECTION ( 'NONE',  ( 0.000000000000000000, 0.000000000000000000, 1.000000000000000000 ) ) ;
#5630=DIRECTION ( 'NONE',  ( -0.000000000000000000, -1.000000000000000000, -0.000000000000000000 ) ) ;
#5632=CARTESIAN_POINT ( 'NONE',  ( 17.40975659021752620, 4.268749999044084475, 17.40975659021753330 ) ) ;
#5638=CARTESIAN_POINT ( 'NONE',  ( 10.19839929293505953, 3.406249999044085097, -24.62111388750000174 ) ) ;
#5640=EDGE_CURVE ( 'NONE', #4321, #9229, #1996, .T. ) ;
#5642=ORIENTED_EDGE ( 'NONE', *, *, #5986, .F. ) ;
#5643=CIRCLE ( 'NONE', #879, 5.999999999999999112 ) ;
#5647=DIRECTION ( 'NONE',  ( 0.4999999999999947820, 0.000000000000000000, -0.8660254037844417052 ) ) ;
#5648=CARTESIAN_POINT ( 'NONE',  ( -10.19839929293505776, 2.531249999044085097, -24.62111388750000174 ) ) ;
#5652=FACE_OUTER_BOUND ( 'NONE', #6527, .T. ) ;
#5655=CIRCLE ( 'NONE', #884, 2.999999999999997335 ) ;
#5658=ORIENTED_EDGE ( 'NONE', *, *, #9019, .F. ) ;
#5659=ORIENTED_EDGE ( 'NONE', *, *, #1576, .F. ) ;
#5663=AXIS2_PLACEMENT_3D ( 'NONE', #10378, #9553, #7306 ) ;
#5665=CARTESIAN_POINT ( 'NONE',  ( -17.10400172474254532, 28.00000000000000000, 12.87500000000020250 ) ) ;
#5670=CIRCLE ( 'NONE', #8480, 2.999999999999998668 ) ;
#5671=ORIENTED_EDGE ( 'NONE', *, *, #5413, .T. ) ;
#5672=ADVANCED_FACE ( 'NONE', ( #5461 ), #380, .F. ) ;
#5673=ORIENTED_EDGE ( 'NONE', *, *, #6268, .T. ) ;
#5674=ORIENTED_EDGE ( 'NONE', *, *, #646, .T. ) ;
#5679=LINE ( 'NONE', #6670, #2346 ) ;
#5680=PLANE ( 'NONE',  #225 ) ;
#5681=ORIENTED_EDGE ( 'NONE', *, *, #5200, .T. ) ;
#5682=AXIS2_PLACEMENT_3D ( 'NONE', #6102, #896, #2706 ) ;
#5683=CARTESIAN_POINT ( 'NONE',  ( 0.000000000000000000, 28.00000000000000000, 0.000000000000000000 ) ) ;
#5684=DIRECTION ( 'NONE',  ( -0.000000000000000000, 1.000000000000000000, -0.000000000000000000 ) ) ;
#5685=CARTESIAN_POINT ( 'NONE',  ( 18.60400172474268032, 28.00000000000000000, 7.276923788646640467 ) ) ;
#5686=CARTESIAN_POINT ( 'NONE',  ( -17.40975659021752975, 2.768749999044084475, -17.40975659021752975 ) ) ;
#5687=ORIENTED_EDGE ( 'NONE', *, *, #9624, .F. ) ;
#5693=CARTESIAN_POINT ( 'NONE',  ( -24.62111388750000174, 0.7187499990440845421, -3.015216831376932151E-15 ) ) ;
#5694=AXIS2_PLACEMENT_3D ( 'NONE', #313, #4478, #5194 ) ;
#5695=VERTEX_POINT ( 'NONE', #7906 ) ;
#5696=ORIENTED_EDGE ( 'NONE', *, *, #8198, .F. ) ;
#5698=CIRCLE ( 'NONE', #6579, 25.00000000000000000 ) ;
#5702=CARTESIAN_POINT ( 'NONE',  ( -24.62111388750000174, 3.718749999044084653, -3.015216831376932151E-15 ) ) ;
#5703=ORIENTED_EDGE ( 'NONE', *, *, #4452, .T. ) ;
#5704=EDGE_CURVE ( 'NONE', #9703, #4100, #8732, .T. ) ;
#5707=VECTOR ( 'NONE', #1549, 1000.000000000000000 ) ;
#5711=CARTESIAN_POINT ( 'NONE',  ( 2.999999999999998224, 25.00000000000000000, 15.75000000000000355 ) ) ;
#5714=VERTEX_POINT ( 'NONE', #2950 ) ;
#5716=EDGE_CURVE ( 'NONE', #1227, #2972, #2871, .T. ) ;
#5718=CARTESIAN_POINT ( 'NONE',  ( 24.62111388750000174, 1.218749999044084431, 0.000000000000000000 ) ) ;
#5726=VERTEX_POINT ( 'NONE', #9710 ) ;
#5727=EDGE_LOOP ( 'NONE', ( #8545, #5946, #8317, #1533 ) ) ;
#5730=DIRECTION ( 'NONE',  ( -0.8660254037844327124, 0.000000000000000000, 0.5000000000000103251 ) ) ;
#5732=DIRECTION ( 'NONE',  ( 0.000000000000000000, 1.000000000000000000, 0.000000000000000000 ) ) ;
#5734=DIRECTION ( 'NONE',  ( 0.000000000000000000, 1.000000000000000000, 0.000000000000000000 ) ) ;
#5735=EDGE_CURVE ( 'NONE', #5067, #2931, #1131, .T. ) ;
#5739=CARTESIAN_POINT ( 'NONE',  ( -24.62111388750000884, 4.956249999044084475, 10.19839929293505421 ) ) ;
#5744=CARTESIAN_POINT ( 'NONE',  ( 17.40975659021752975, 2.343749999044085097, -17.40975659021752975 ) ) ;
#5745=VERTEX_POINT ( 'NONE', #9659 ) ;
#5748=CARTESIAN_POINT ( 'NONE',  ( 10.19839929293506486, 2.031249999044084653, 24.62111388749999819 ) ) ;
#5752=DIRECTION ( 'NONE',  ( 0.000000000000000000, 1.000000000000000000, 0.000000000000000000 ) ) ;
#5755=CARTESIAN_POINT ( 'NONE',  ( 3.061616997868383043E-15, 85.00000000000000000, 25.00000000000000000 ) ) ;
#5757=EDGE_LOOP ( 'NONE', ( #2493, #3600, #9801, #7693, #3321 ) ) ;
#5758=CARTESIAN_POINT ( 'NONE',  ( 24.62111388750000174, 2.456249999044084475, -10.19839929293505776 ) ) ;
#5764=CARTESIAN_POINT ( 'NONE',  ( 7.874999999999916511, 28.00000000000000000, -13.63990010960495702 ) ) ;
#5770=VERTEX_POINT ( 'NONE', #5835 ) ;
#5772=ORIENTED_EDGE ( 'NONE', *, *, #9277, .F. ) ;
#5775=VECTOR ( 'NONE', #6210, 1000.000000000000000 ) ;
#5777=( BOUNDED_CURVE ( )  B_SPLINE_CURVE ( 2, ( #1050, #7667, #157, #97, #3455 ),
 .UNSPECIFIED., .F., .F. ) 
 B_SPLINE_CURVE_WITH_KNOTS ( ( 3, 2, 3 ),
 ( 0.9500000000000000666, 0.9750000000000000888, 1.000000000000000000 ),
 .UNSPECIFIED. ) 
 CURVE ( )  GEOMETRIC_REPRESENTATION_ITEM ( )  RATIONAL_B_SPLINE_CURVE ( ( 0.9999999999999996669, 0.9238795325112870716, 1.000000000000000000, 0.9238795325112867385, 1.000000000000000000 ) ) 
 REPRESENTATION_ITEM ( '' )  );
#5784=VERTEX_POINT ( 'NONE', #8255 ) ;
#5785=VERTEX_POINT ( 'NONE', #1476 ) ;
#5793=VERTEX_POINT ( 'NONE', #4077 ) ;
#5796=CARTESIAN_POINT ( 'NONE',  ( -10.19839929293505776, 0.5312499990440845421, -24.62111388750000174 ) ) ;
#5798=ORIENTED_EDGE ( 'NONE', *, *, #5716, .T. ) ;
#5799=EDGE_CURVE ( 'NONE', #2242, #2252, #5148, .T. ) ;
#5802=CARTESIAN_POINT ( 'NONE',  ( -24.62111388750000884, 1.781249999044084431, 10.19839929293505421 ) ) ;
#5808=DIRECTION ( 'NONE',  ( -0.000000000000000000, 1.000000000000000000, -0.000000000000000000 ) ) ;
#5810=PLANE ( 'NONE',  #8683 ) ;
#5811=PLANE ( 'NONE',  #2979 ) ;
#5812=VERTEX_POINT ( 'NONE', #3218 ) ;
#5813=ORIENTED_EDGE ( 'NONE', *, *, #4473, .T. ) ;
#5814=CARTESIAN_POINT ( 'NONE',  ( 10.35533905932738286, 5.424999998088169129, 24.99999999999999645 ) ) ;
#5821=DIRECTION ( 'NONE',  ( 0.000000000000000000, 0.000000000000000000, 1.000000000000000000 ) ) ;
#5822=LINE ( 'NONE', #1734, #1801 ) ;
#5825=ORIENTED_EDGE ( 'NONE', *, *, #6080, .T. ) ;
#5827=AXIS2_PLACEMENT_3D ( 'NONE', #3510, #9488, #4539 ) ;
#5829=VERTEX_POINT ( 'NONE', #8984 ) ;
#5830=PLANE ( 'NONE',  #8323 ) ;
#5831=EDGE_CURVE ( 'NONE', #6402, #1429, #3655, .T. ) ;
#5832=DIRECTION ( 'NONE',  ( -2.168404344971010594E-16, 0.000000000000000000, -1.000000000000000000 ) ) ;
#5834=AXIS2_PLACEMENT_3D ( 'NONE', #3397, #10876, #1645 ) ;
#5835=CARTESIAN_POINT ( 'NONE',  ( -15.13990010960484867, 28.00000000000000000, 5.276923788646865177 ) ) ;
#5837=EDGE_CURVE ( 'NONE', #7237, #5856, #3945, .T. ) ;
#5840=CARTESIAN_POINT ( 'NONE',  ( 15.75000000000001421, 25.00000000000000000, 2.999999999999942268 ) ) ;
#5845=ORIENTED_EDGE ( 'NONE', *, *, #10086, .T. ) ;
#5846=EDGE_CURVE ( 'NONE', #2468, #7557, #5679, .T. ) ;
#5851=CARTESIAN_POINT ( 'NONE',  ( 0.000000000000000000, 31.00000000000000000, -7.500000000000000888 ) ) ;
#5852=CARTESIAN_POINT ( 'NONE',  ( 17.40975659021752620, 2.093749999044084653, 17.40975659021753330 ) ) ;
#5853=ADVANCED_FACE ( 'NONE', ( #3163, #2354 ), #6559, .T. ) ;
#5855=VECTOR ( 'NONE', #7349, 1000.000000000000000 ) ;
#5856=VERTEX_POINT ( 'NONE', #4236 ) ;
#5857=VECTOR ( 'NONE', #6206, 1000.000000000000000 ) ;
#5859=CARTESIAN_POINT ( 'NONE',  ( -7.875000000000116351, -0.001000000000001000089, -10.63990010960484511 ) ) ;
#5860=CARTESIAN_POINT ( 'NONE',  ( 24.62111388749999463, 3.156249999044084653, 10.19839929293507730 ) ) ;
#5866=AXIS2_PLACEMENT_3D ( 'NONE', #2893, #3738, #5304 ) ;
#5867=CARTESIAN_POINT ( 'NONE',  ( 9.184850993605149917E-16, 28.00000000000000000, 7.500000000000000888 ) ) ;
#5873=EDGE_CURVE ( 'NONE', #5829, #9988, #10926, .T. ) ;
#5878=FACE_OUTER_BOUND ( 'NONE', #6599, .T. ) ;
#5879=CARTESIAN_POINT ( 'NONE',  ( 17.40975659021752620, 3.268749999044084475, 17.40975659021753330 ) ) ;
#5880=AXIS2_PLACEMENT_3D ( 'NONE', #2181, #3733, #7932 ) ;
#5881=CARTESIAN_POINT ( 'NONE',  ( -24.62111388750000174, 1.718749999044084431, -3.015216831376932151E-15 ) ) ;
#5891=VECTOR ( 'NONE', #8764, 999.9999999999998863 ) ;
#5894=EDGE_LOOP ( 'NONE', ( #4014, #1130, #6370, #1594 ) ) ;
#5895=AXIS2_PLACEMENT_3D ( 'NONE', #6975, #8607, #4646 ) ;
#5900=CARTESIAN_POINT ( 'NONE',  ( -3.223142256880076948E-15, 25.00000000000000000, -12.75000000000000178 ) ) ;
#5904=DIRECTION ( 'NONE',  ( 0.000000000000000000, 0.000000000000000000, -1.000000000000000000 ) ) ;
#5910=CARTESIAN_POINT ( 'NONE',  ( 0.000000000000000000, 85.00000000000000000, 0.000000000000000000 ) ) ;
#5912=ADVANCED_FACE ( 'NONE', ( #3388 ), #6252, .F. ) ;
#5918=FACE_OUTER_BOUND ( 'NONE', #4188, .T. ) ;
#5927=EDGE_CURVE ( 'NONE', #2102, #2070, #3327, .T. ) ;
#5928=ORIENTED_EDGE ( 'NONE', *, *, #8553, .F. ) ;
#5933=CARTESIAN_POINT ( 'NONE',  ( -24.62111388750000884, 1.956249999044084475, 10.19839929293505421 ) ) ;
#5934=CARTESIAN_POINT ( 'NONE',  ( -10.35533905932739174, 0.6875000000000000000, 24.99999999999999289 ) ) ;
#5935=ADVANCED_FACE ( 'NONE', ( #149 ), #9432, .F. ) ;
#5945=DIRECTION ( 'NONE',  ( 0.8660254037844434816, 0.000000000000000000, 0.4999999999999918399 ) ) ;
#5946=ORIENTED_EDGE ( 'NONE', *, *, #398, .T. ) ;
#5949=CARTESIAN_POINT ( 'NONE',  ( -12.47307621135344391, -0.001000000000001000089, -15.60400172474256131 ) ) ;
#5950=FACE_OUTER_BOUND ( 'NONE', #965, .T. ) ;
#5951=LINE ( 'NONE', #92, #3377 ) ;
#5956=DIRECTION ( 'NONE',  ( -0.000000000000000000, 1.000000000000000000, -0.000000000000000000 ) ) ;
#5959=EDGE_LOOP ( 'NONE', ( #6721, #7807, #783, #3482 ) ) ;
#5965=CARTESIAN_POINT ( 'NONE',  ( 0.000000000000000000, 31.00000000000000000, 0.000000000000000000 ) ) ;
#5966=VECTOR ( 'NONE', #4157, 1000.000000000000000 ) ;
#5968=VERTEX_POINT ( 'NONE', #3509 ) ;
#5972=CIRCLE ( 'NONE', #4403, 2.999999999999997335 ) ;
#5982=( BOUNDED_CURVE ( )  B_SPLINE_CURVE ( 2, ( #234, #2701, #10219, #1947, #3532, #6751, #7801, #7741, #5154 ),
 .UNSPECIFIED., .F., .F. ) 
 B_SPLINE_CURVE_WITH_KNOTS ( ( 3, 2, 2, 2, 3 ),
 ( 0.05000000000000000278, 0.07499999999999999722, 0.1000000000000000056, 0.1250000000000000000, 0.1499999999999999944 ),
 .UNSPECIFIED. ) 
 CURVE ( )  GEOMETRIC_REPRESENTATION_ITEM ( )  RATIONAL_B_SPLINE_CURVE ( ( 1.000000000000000000, 0.9238795325112867385, 1.000000000000000000, 0.9238795325112867385, 1.000000000000000000, 0.9238795325112867385, 1.000000000000000000, 0.9238795325112867385, 1.000000000000000000 ) ) 
 REPRESENTATION_ITEM ( '' )  );
#5983=AXIS2_PLACEMENT_3D ( 'NONE', #968, #3485, #10460 ) ;
#5985=ORIENTED_EDGE ( 'NONE', *, *, #6957, .F. ) ;
#5986=EDGE_CURVE ( 'NONE', #849, #4742, #1303, .T. ) ;
#5989=CARTESIAN_POINT ( 'NONE',  ( 24.62111388750000174, 0.3937499990440845865, 0.000000000000000000 ) ) ;
#5990=CARTESIAN_POINT ( 'NONE',  ( -10.19839929293505776, 1.706249999044084698, -24.62111388750000174 ) ) ;
#5991=CARTESIAN_POINT ( 'NONE',  ( 1.507608415688466075E-15, 3.468749999044085097, -24.62111388750000174 ) ) ;
#5992=FACE_OUTER_BOUND ( 'NONE', #612, .T. ) ;
#5993=EDGE_CURVE ( 'NONE', #3078, #1567, #2694, .T. ) ;
#6002=ADVANCED_FACE ( 'NONE', ( #4538 ), #2782, .T. ) ;
#6003=DIRECTION ( 'NONE',  ( 1.156482317317872514E-15, 0.000000000000000000, 1.000000000000000000 ) ) ;
#6004=AXIS2_PLACEMENT_3D ( 'NONE', #6224, #4524, #5398 ) ;
#6009=DIRECTION ( 'NONE',  ( 0.000000000000000000, 1.000000000000000000, 0.000000000000000000 ) ) ;
#6011=DIRECTION ( 'NONE',  ( -0.000000000000000000, -1.000000000000000000, -0.000000000000000000 ) ) ;
#6018=DIRECTION ( 'NONE',  ( -0.000000000000000000, 1.000000000000000000, -0.000000000000000000 ) ) ;
#6023=DIRECTION ( 'NONE',  ( 0.4999999999999887312, 0.000000000000000000, -0.8660254037844451469 ) ) ;
#6026=CARTESIAN_POINT ( 'NONE',  ( -10.19839929293507375, 4.906249999044083765, 24.62111388749999108 ) ) ;
#6030=CARTESIAN_POINT ( 'NONE',  ( -2.999999999999997335, 25.00000000000000000, 15.75000000000000355 ) ) ;
#6031=CARTESIAN_POINT ( 'NONE',  ( 0.000000000000000000, 85.00000000000000000, -25.00000000000000000 ) ) ;
#6040=CIRCLE ( 'NONE', #3368, 2.999999999999997780 ) ;
#6044=VERTEX_POINT ( 'NONE', #8655 ) ;
#6045=DIRECTION ( 'NONE',  ( -0.000000000000000000, 1.000000000000000000, -0.000000000000000000 ) ) ;
#6047=VECTOR ( 'NONE', #7312, 1000.000000000000000 ) ;
#6049=CARTESIAN_POINT ( 'NONE',  ( 17.67766952966368521, 4.487499998088169129, 17.67766952966369232 ) ) ;
#6050=CARTESIAN_POINT ( 'NONE',  ( -10.35533905932737575, 0.3125000000000000000, -25.00000000000000000 ) ) ;
#6051=ORIENTED_EDGE ( 'NONE', *, *, #1541, .F. ) ;
#6053=FACE_BOUND ( 'NONE', #4811, .T. ) ;
#6054=FACE_OUTER_BOUND ( 'NONE', #5959, .T. ) ;
#6057=AXIS2_PLACEMENT_3D ( 'NONE', #3625, #5300, #4349 ) ;
#6058=VERTEX_POINT ( 'NONE', #6125 ) ;
#6059=CIRCLE ( 'NONE', #2681, 10.50000000000000000 ) ;
#6060=ORIENTED_EDGE ( 'NONE', *, *, #3846, .F. ) ;
#6062=ORIENTED_EDGE ( 'NONE', *, *, #7325, .F. ) ;
#6068=AXIS2_PLACEMENT_3D ( 'NONE', #8043, #1404, #475 ) ;
#6069=CARTESIAN_POINT ( 'NONE',  ( 13.63990010960487353, 28.00000000000000000, -7.875000000000067502 ) ) ;
#6077=CARTESIAN_POINT ( 'NONE',  ( 10.19839929293505953, 4.581249999044083587, -24.62111388750000174 ) ) ;
#6079=CIRCLE ( 'NONE', #5532, 5.999999999999999112 ) ;
#6080=EDGE_CURVE ( 'NONE', #7345, #3125, #6414, .T. ) ;
#6082=AXIS2_PLACEMENT_3D ( 'NONE', #8040, #1307, #6545 ) ;
#6086=DIRECTION ( 'NONE',  ( 1.000000000000000000, 0.000000000000000000, -3.708321773340234242E-15 ) ) ;
#6087=ADVANCED_FACE ( 'NONE', ( #833 ), #2473, .F. ) ;
#6090=CARTESIAN_POINT ( 'NONE',  ( 24.62111388750000174, 4.281249999044084653, -10.19839929293505776 ) ) ;
#6094=CARTESIAN_POINT ( 'NONE',  ( -24.62111388750000174, 4.656249999044085541, -10.19839929293506131 ) ) ;
#6095=CARTESIAN_POINT ( 'NONE',  ( -17.40975659021752975, 1.768749999044084475, -17.40975659021752975 ) ) ;
#6097=CARTESIAN_POINT ( 'NONE',  ( 13.63990010960492860, 25.00000000000000000, 7.874999999999965361 ) ) ;
#6099=CARTESIAN_POINT ( 'NONE',  ( 1.530808498934191521E-15, 1.862499998088169129, -25.00000000000000000 ) ) ;
#6100=FACE_OUTER_BOUND ( 'NONE', #8245, .T. ) ;
#6102=CARTESIAN_POINT ( 'NONE',  ( -13.63990010960481492, 25.00000000000000000, 7.875000000000163425 ) ) ;
#6108=CARTESIAN_POINT ( 'NONE',  ( 0.000000000000000000, 31.00000000000000000, 0.000000000000000000 ) ) ;
#6109=CARTESIAN_POINT ( 'NONE',  ( 24.99999999999999289, 2.549999998088169129, 10.35533905932739529 ) ) ;
#6110=CARTESIAN_POINT ( 'NONE',  ( -17.40975659021753330, 2.843749999044085097, 17.40975659021752975 ) ) ;
#6111=( NAMED_UNIT ( * ) SI_UNIT ( $, .STERADIAN. ) SOLID_ANGLE_UNIT ( ) );
#6118=ORIENTED_EDGE ( 'NONE', *, *, #10232, .F. ) ;
#6120=VERTEX_POINT ( 'NONE', #9324 ) ;
#6123=CYLINDRICAL_SURFACE ( 'NONE', #4501, 2.999999999999997780 ) ;
#6125=CARTESIAN_POINT ( 'NONE',  ( 2.999999999999996447, 25.00000000000000000, -19.75000000000000000 ) ) ;
#6127=CARTESIAN_POINT ( 'NONE',  ( 7.874999999999916511, 25.00000000000000000, -13.63990010960495702 ) ) ;
#6130=EDGE_CURVE ( 'NONE', #4742, #7447, #2422, .T. ) ;
#6136=CYLINDRICAL_SURFACE ( 'NONE', #5895, 2.999999999999999112 ) ;
#6139=CARTESIAN_POINT ( 'NONE',  ( -15.60400172474251868, -0.001000000000001000089, 12.47307621135349720 ) ) ;
#6142=LINE ( 'NONE', #9509, #7958 ) ;
#6144=CARTESIAN_POINT ( 'NONE',  ( -17.40975659021752975, 4.593749999044084653, -17.40975659021752975 ) ) ;
#6147=DIRECTION ( 'NONE',  ( 0.5000000000000103251, 0.000000000000000000, 0.8660254037844327124 ) ) ;
#6148=CARTESIAN_POINT ( 'NONE',  ( 15.74999999999999289, -0.001000000000001000089, -3.000000000000055955 ) ) ;
#6150=CARTESIAN_POINT ( 'NONE',  ( -13.63990010960498367, -0.001000000000001000089, -7.874999999999870326 ) ) ;
#6152=ORIENTED_EDGE ( 'NONE', *, *, #5873, .T. ) ;
#6154=EDGE_LOOP ( 'NONE', ( #4053, #6801 ) ) ;
#6162=CARTESIAN_POINT ( 'NONE',  ( -10.35533905932737575, 2.924999998088168685, -25.00000000000000000 ) ) ;
#6163=CARTESIAN_POINT ( 'NONE',  ( -24.62111388750000174, 4.656249999044085541, -10.19839929293506131 ) ) ;
#6164=DIRECTION ( 'NONE',  ( -0.000000000000000000, 1.000000000000000000, -0.000000000000000000 ) ) ;
#6166=FACE_OUTER_BOUND ( 'NONE', #1844, .T. ) ;
#6167=DIRECTION ( 'NONE',  ( 0.000000000000000000, 1.000000000000000000, -0.000000000000000000 ) ) ;
#6169=AXIS2_PLACEMENT_3D ( 'NONE', #3654, #238, #2756 ) ;
#6171=FACE_OUTER_BOUND ( 'NONE', #179, .T. ) ;
#6172=ORIENTED_EDGE ( 'NONE', *, *, #9031, .T. ) ;
#6175=DIRECTION ( 'NONE',  ( 0.000000000000000000, 1.000000000000000000, 0.000000000000000000 ) ) ;
#6176=CARTESIAN_POINT ( 'NONE',  ( 24.81055694375000087, 0.1093749995220422710, 0.000000000000000000 ) ) ;
#6180=CARTESIAN_POINT ( 'NONE',  ( 1.530808498934191521E-15, 1.862499998088169129, -25.00000000000000000 ) ) ;
#6181=CARTESIAN_POINT ( 'NONE',  ( -24.62111388750000174, 4.831249999044084475, -10.19839929293506131 ) ) ;
#6185=ORIENTED_EDGE ( 'NONE', *, *, #9748, .F. ) ;
#6192=DIRECTION ( 'NONE',  ( -0.000000000000000000, 1.000000000000000000, -0.000000000000000000 ) ) ;
#6193=CARTESIAN_POINT ( 'NONE',  ( 13.63990010960487353, 25.00000000000000000, -7.875000000000067502 ) ) ;
#6197=ADVANCED_FACE ( 'NONE', ( #8501 ), #3352, .T. ) ;
#6199=AXIS2_PLACEMENT_3D ( 'NONE', #4626, #7054, #5237 ) ;
#6202=ADVANCED_FACE ( 'NONE', ( #8559 ), #6749, .F. ) ;
#6205=CARTESIAN_POINT ( 'NONE',  ( -25.00000000000000000, 0.4374999999999999445, -10.35533905932738108 ) ) ;
#6206=DIRECTION ( 'NONE',  ( -0.000000000000000000, -1.000000000000000000, -0.000000000000000000 ) ) ;
#6210=DIRECTION ( 'NONE',  ( 0.000000000000000000, 1.000000000000000000, 0.000000000000000000 ) ) ;
#6212=VECTOR ( 'NONE', #1855, 1000.000000000000000 ) ;
#6213=AXIS2_PLACEMENT_3D ( 'NONE', #9022, #8295, #736 ) ;
#6214=ORIENTED_EDGE ( 'NONE', *, *, #10430, .T. ) ;
#6219=CARTESIAN_POINT ( 'NONE',  ( -4.522825247065398226E-15, 4.143749999044084475, 24.62111388750000174 ) ) ;
#6220=CARTESIAN_POINT ( 'NONE',  ( -17.67766952966369232, 2.237499998088169573, 17.67766952966368876 ) ) ;
#6221=CARTESIAN_POINT ( 'NONE',  ( -17.67766952966368876, 1.375000000000000000, -17.67766952966369232 ) ) ;
#6222=( NAMED_UNIT ( * ) PLANE_ANGLE_UNIT ( ) SI_UNIT ( $, .RADIAN. ) );
#6223=CIRCLE ( 'NONE', #4458, 2.999999999999997335 ) ;
#6224=CARTESIAN_POINT ( 'NONE',  ( 9.875000000000023093, 25.00000000000000000, 17.10400172474264835 ) ) ;
#6226=CARTESIAN_POINT ( 'NONE',  ( 18.60400172474263414, -0.001000000000001000089, -7.276923788646775471 ) ) ;
#6231=CIRCLE ( 'NONE', #4470, 2.999999999999996891 ) ;
#6232=EDGE_LOOP ( 'NONE', ( #8688, #8760, #4451, #3715, #7194 ) ) ;
#6234=VECTOR ( 'NONE', #9768, 1000.000000000000000 ) ;
#6237=CARTESIAN_POINT ( 'NONE',  ( -12.47307621135311351, 25.00000000000000000, 15.60400172474282599 ) ) ;
#6238=AXIS2_PLACEMENT_3D ( 'NONE', #7429, #9304, #4133 ) ;
#6240=AXIS2_PLACEMENT_3D ( 'NONE', #5077, #867, #4237 ) ;
#6244=CARTESIAN_POINT ( 'NONE',  ( -24.62111388750000174, 4.893749999044084475, -3.015216831376932151E-15 ) ) ;
#6246=AXIS2_PLACEMENT_3D ( 'NONE', #9397, #6985, #5327 ) ;
#6251=CARTESIAN_POINT ( 'NONE',  ( 0.000000000000000000, 20.00000000000000355, 0.000000000000000000 ) ) ;
#6252=CONICAL_SURFACE ( 'NONE', #9051, 20.00000000000000000, 0.3947911196997613281 ) ;
#6258=CARTESIAN_POINT ( 'NONE',  ( -17.67766952966369232, 0.6250000000000000000, 17.67766952966368876 ) ) ;
#6259=CARTESIAN_POINT ( 'NONE',  ( 24.62111388750000174, 0.3937499990440845310, 0.000000000000000000 ) ) ;
#6263=LINE ( 'NONE', #392, #3034 ) ;
#6265=CARTESIAN_POINT ( 'NONE',  ( 10.35533905932737930, 2.799999998088169573, -25.00000000000000000 ) ) ;
#6266=ADVANCED_FACE ( 'NONE', ( #5918 ), #5091, .F. ) ;
#6268=EDGE_CURVE ( 'NONE', #5295, #3918, #339, .T. ) ;
#6269=ORIENTED_EDGE ( 'NONE', *, *, #7200, .T. ) ;
#6274=CARTESIAN_POINT ( 'NONE',  ( -24.62111388750000174, 4.893749999044085364, -3.015216831376932151E-15 ) ) ;
#6275=CARTESIAN_POINT ( 'NONE',  ( 25.00000000000000000, 3.000000000000000000, 0.000000000000000000 ) ) ;
#6280=EDGE_CURVE ( 'NONE', #2862, #7767, #7912, .T. ) ;
#6285=( BOUNDED_CURVE ( )  B_SPLINE_CURVE ( 2, ( #4681, #8032, #8132, #10568, #2977, #8960, #6385, #9736, #2169 ),
 .UNSPECIFIED., .F., .F. ) 
 B_SPLINE_CURVE_WITH_KNOTS ( ( 3, 2, 2, 2, 3 ),
 ( 0.1500000000000000222, 0.1750000000000000167, 0.2000000000000000389, 0.2250000000000000333, 0.2500000000000000000 ),
 .UNSPECIFIED. ) 
 CURVE ( )  GEOMETRIC_REPRESENTATION_ITEM ( )  RATIONAL_B_SPLINE_CURVE ( ( 0.9999999999999998890, 0.9238795325112868495, 1.000000000000000000, 0.9238795325112867385, 1.000000000000000000, 0.9238795325112867385, 1.000000000000000000, 0.9238795325112867385, 1.000000000000000000 ) ) 
 REPRESENTATION_ITEM ( '' )  );
#6288=DIRECTION ( 'NONE',  ( 0.000000000000000000, 0.000000000000000000, 1.000000000000000000 ) ) ;
#6289=CARTESIAN_POINT ( 'NONE',  ( 12.47307621135333200, 28.00000000000000000, 15.60400172474264835 ) ) ;
#6295=ORIENTED_EDGE ( 'NONE', *, *, #2735, .F. ) ;
#6298=CARTESIAN_POINT ( 'NONE',  ( 5.276923788646596947, 28.00000000000000000, -15.13990010960494459 ) ) ;
#6300=CARTESIAN_POINT ( 'NONE',  ( -17.10400172474254532, -0.001000000000001000089, 9.875000000000202505 ) ) ;
#6302=DIRECTION ( 'NONE',  ( 2.168404344971010347E-16, 0.000000000000000000, 1.000000000000000000 ) ) ;
#6303=FACE_OUTER_BOUND ( 'NONE', #10836, .T. ) ;
#6305=EDGE_LOOP ( 'NONE', ( #2432, #1277, #9054, #4670, #5545 ) ) ;
#6306=CARTESIAN_POINT ( 'NONE',  ( 1.530808498934191521E-15, 0.8624999980881691286, -25.00000000000000000 ) ) ;
#6310=CARTESIAN_POINT ( 'NONE',  ( 0.000000000000000000, 20.00000000000000355, 0.000000000000000000 ) ) ;
#6318=CARTESIAN_POINT ( 'NONE',  ( -10.19839929293505776, 3.706249999044084920, -24.62111388750000174 ) ) ;
#6321=CARTESIAN_POINT ( 'NONE',  ( -25.00000000000001421, 4.562500000000000888, 10.35533905932737397 ) ) ;
#6326=CARTESIAN_POINT ( 'NONE',  ( 7.276923788646707969, -0.001000000000001000089, 18.60400172474265190 ) ) ;
#6327=( GEOMETRIC_REPRESENTATION_CONTEXT ( 3 ) GLOBAL_UNCERTAINTY_ASSIGNED_CONTEXT ( ( #6707 ) ) GLOBAL_UNIT_ASSIGNED_CONTEXT ( ( #3665, #6222, #6111 ) ) REPRESENTATION_CONTEXT ( 'NONE', 'WORKASPACE' ) );
#6331=ORIENTED_EDGE ( 'NONE', *, *, #4234, .T. ) ;
#6332=ORIENTED_EDGE ( 'NONE', *, *, #5986, .T. ) ;
#6333=EDGE_LOOP ( 'NONE', ( #8661, #8304, #305, #3565 ) ) ;
#6338=AXIS2_PLACEMENT_3D ( 'NONE', #6991, #6, #10126 ) ;
#6340=LINE ( 'NONE', #6289, #5891 ) ;
#6342=CARTESIAN_POINT ( 'NONE',  ( 13.63990010960487353, 28.00000000000000000, -7.875000000000067502 ) ) ;
#6345=( BOUNDED_SURFACE ( )  B_SPLINE_SURFACE ( 1, 2, ( 
 ( #5989, #5169, #3545, #8517, #970, #2647, #4334, #7697, #4391, #7753, #6939, #10298, #6431, #10463, #4718, #3939, #7243, #2106, #3875, #7151, #5484, #3722, #456, #10614, #9731, #6377, #8797, #5593, #7193, #7974, #3779, #504, #406, #2161, #4768, #7100, #3031, #9781, #5544, #8123, #10672, #10515, #2058, #2213, #8748, #8904, #5435, #8953, #2971, #1339, #2920, #9580, #8848, #6318, #8071, #1383, #554, #9683, #7296, #1292, #6219, #4675, #2020, #5392, #10561, #3826, #1187, #4568, #2877, #4619, #1236, #7922, #6274, #8025, #350, #9631, #9066, #1661, #9882, #3183, #611 ),
 ( #8339, #6695, #5041, #2421, #8225, #4877, #9165, #2373, #7511, #4044, #832, #7562, #9831, #665, #10777, #7398, #781, #6583, #4826, #6476, #10834, #9942, #2317, #3992, #3083, #5802, #10051, #4151, #9218, #5748, #1599, #8182, #2264, #3234, #4985, #7457, #8388, #5648, #4099, #4200, #9006, #9110, #10890, #3292, #2472, #6633, #1545, #5860, #1432, #7344, #4929, #9991, #8277, #720, #10719, #3132, #5702, #6526, #1496, #1708, #9454, #1943, #6923, #10281, #2750, #3468, #2526, #3351, #2698, #4437, #6144, #6094, #9511, #1886, #7738, #8441, #231, #954, #5265, #5321, #1834 ) ),
 .UNSPECIFIED., .F., .F., .F. ) 
 B_SPLINE_SURFACE_WITH_KNOTS ( ( 2, 2 ),
 ( 3, 2, 2, 2, 2, 2, 2, 2, 2, 2, 2, 2, 2, 2, 2, 2, 2, 2, 2, 2, 2, 2, 2, 2, 2, 2, 2, 2, 2, 2, 2, 2, 2, 2, 2, 2, 2, 2, 2, 2, 3 ),
 ( 0.000000000000000000, 1.000000000000000000 ),
 ( 0.000000000000000000, 0.02500000000000000139, 0.05000000000000000278, 0.07499999999999999722, 0.1000000000000000056, 0.1250000000000000000, 0.1499999999999999944, 0.1749999999999999889, 0.2000000000000000111, 0.2250000000000000056, 0.2500000000000000000, 0.2750000000000000222, 0.2999999999999999889, 0.3250000000000000111, 0.3499999999999999778, 0.3750000000000000000, 0.4000000000000000222, 0.4249999999999999889, 0.4500000000000000111, 0.4749999999999999778, 0.5000000000000000000, 0.5250000000000000222, 0.5500000000000000444, 0.5749999999999999556, 0.5999999999999999778, 0.6250000000000000000, 0.6500000000000000222, 0.6750000000000000444, 0.6999999999999999556, 0.7249999999999999778, 0.7500000000000000000, 0.7750000000000000222, 0.8000000000000000444, 0.8249999999999999556, 0.8499999999999999778, 0.8750000000000000000, 0.9000000000000000222, 0.9250000000000000444, 0.9499999999999999556, 0.9749999999999999778, 1.000000000000000000 ),
 .UNSPECIFIED. ) 
 GEOMETRIC_REPRESENTATION_ITEM ( )  RATIONAL_B_SPLINE_SURFACE ( (
 ( 1.000000000000000000, 0.9238795325112867385, 1.000000000000000000, 0.9238795325112867385, 1.000000000000000000, 0.9238795325112867385, 1.000000000000000000, 0.9238795325112867385, 1.000000000000000000, 0.9238795325112867385, 1.000000000000000000, 0.9238795325112867385, 1.000000000000000000, 0.9238795325112867385, 1.000000000000000000, 0.9238795325112867385, 1.000000000000000000, 0.9238795325112867385, 1.000000000000000000, 0.9238795325112867385, 1.000000000000000000, 0.9238795325112867385, 1.000000000000000000, 0.9238795325112867385, 1.000000000000000000, 0.9238795325112867385, 1.000000000000000000, 0.9238795325112867385, 1.000000000000000000, 0.9238795325112867385, 1.000000000000000000, 0.9238795325112867385, 1.000000000000000000, 0.9238795325112867385, 1.000000000000000000, 0.9238795325112867385, 1.000000000000000000, 0.9238795325112867385, 1.000000000000000000, 0.9238795325112867385, 1.000000000000000000, 0.9238795325112867385, 1.000000000000000000, 0.9238795325112867385, 1.000000000000000000, 0.9238795325112867385, 1.000000000000000000, 0.9238795325112867385, 1.000000000000000000, 0.9238795325112867385, 1.000000000000000000, 0.9238795325112867385, 1.000000000000000000, 0.9238795325112867385, 1.000000000000000000, 0.9238795325112867385, 1.000000000000000000, 0.9238795325112867385, 1.000000000000000000, 0.9238795325112867385, 1.000000000000000000, 0.9238795325112867385, 1.000000000000000000, 0.9238795325112867385, 1.000000000000000000, 0.9238795325112867385, 1.000000000000000000, 0.9238795325112867385, 1.000000000000000000, 0.9238795325112867385, 1.000000000000000000, 0.9238795325112867385, 1.000000000000000000, 0.9238795325112867385, 1.000000000000000000, 0.9238795325112867385, 1.000000000000000000, 0.9238795325112867385, 1.000000000000000000, 0.9238795325112867385, 1.000000000000000000),
 ( 1.000000000000000000, 0.9238795325112867385, 1.000000000000000000, 0.9238795325112867385, 1.000000000000000000, 0.9238795325112867385, 1.000000000000000000, 0.9238795325112867385, 1.000000000000000000, 0.9238795325112867385, 1.000000000000000000, 0.9238795325112867385, 1.000000000000000000, 0.9238795325112867385, 1.000000000000000000, 0.9238795325112867385, 1.000000000000000000, 0.9238795325112867385, 1.000000000000000000, 0.9238795325112867385, 1.000000000000000000, 0.9238795325112867385, 1.000000000000000000, 0.9238795325112867385, 1.000000000000000000, 0.9238795325112867385, 1.000000000000000000, 0.9238795325112867385, 1.000000000000000000, 0.9238795325112867385, 1.000000000000000000, 0.9238795325112867385, 1.000000000000000000, 0.9238795325112867385, 1.000000000000000000, 0.9238795325112867385, 1.000000000000000000, 0.9238795325112867385, 1.000000000000000000, 0.9238795325112867385, 1.000000000000000000, 0.9238795325112867385, 1.000000000000000000, 0.9238795325112867385, 1.000000000000000000, 0.9238795325112867385, 1.000000000000000000, 0.9238795325112867385, 1.000000000000000000, 0.9238795325112867385, 1.000000000000000000, 0.9238795325112867385, 1.000000000000000000, 0.9238795325112867385, 1.000000000000000000, 0.9238795325112867385, 1.000000000000000000, 0.9238795325112867385, 1.000000000000000000, 0.9238795325112867385, 1.000000000000000000, 0.9238795325112867385, 1.000000000000000000, 0.9238795325112867385, 1.000000000000000000, 0.9238795325112867385, 1.000000000000000000, 0.9238795325112867385, 1.000000000000000000, 0.9238795325112867385, 1.000000000000000000, 0.9238795325112867385, 1.000000000000000000, 0.9238795325112867385, 1.000000000000000000, 0.9238795325112867385, 1.000000000000000000, 0.9238795325112867385, 1.000000000000000000, 0.9238795325112867385, 1.000000000000000000) ) ) 
 REPRESENTATION_ITEM ( '' )  SURFACE ( )  );
#6348=DIRECTION ( 'NONE',  ( -1.000000000000000000, 0.000000000000000000, 1.047444401652940322E-14 ) ) ;
#6349=CARTESIAN_POINT ( 'NONE',  ( -17.10400172474254532, 25.00000000000000000, 12.87500000000020250 ) ) ;
#6350=EDGE_CURVE ( 'NONE', #2070, #10673, #3725, .T. ) ;
#6353=PRODUCT_DEFINITION_FORMATION_WITH_SPECIFIED_SOURCE ( 'ANY', '', #451, .NOT_KNOWN. ) ;
#6356=AXIS2_PLACEMENT_3D ( 'NONE', #6808, #10114, #892 ) ;
#6358=DIRECTION ( 'NONE',  ( 1.000000000000000000, 0.000000000000000000, -3.491481338843131383E-15 ) ) ;
#6361=CARTESIAN_POINT ( 'NONE',  ( 17.40975659021752620, 5.268749999044085364, 17.40975659021753330 ) ) ;
#6362=ORIENTED_EDGE ( 'NONE', *, *, #8832, .F. ) ;
#6370=ORIENTED_EDGE ( 'NONE', *, *, #8806, .T. ) ;
#6374=ORIENTED_EDGE ( 'NONE', *, *, #9156, .F. ) ;
#6377=CARTESIAN_POINT ( 'NONE',  ( -24.62111388750000884, 1.956249999044084475, 10.19839929293505421 ) ) ;
#6378=CARTESIAN_POINT ( 'NONE',  ( 17.67766952966369232, 2.125000000000000000, -17.67766952966369232 ) ) ;
#6382=CARTESIAN_POINT ( 'NONE',  ( 13.63990010960487353, 25.00000000000000000, -4.875000000000069278 ) ) ;
#6383=CARTESIAN_POINT ( 'NONE',  ( 10.35533905932737930, 1.799999998088168907, -25.00000000000000000 ) ) ;
#6384=CYLINDRICAL_SURFACE ( 'NONE', #7806, 2.999999999999999112 ) ;
#6385=CARTESIAN_POINT ( 'NONE',  ( 17.67766952966369232, 1.125000000000000222, -17.67766952966369232 ) ) ;
#6387=ORIENTED_EDGE ( 'NONE', *, *, #3962, .T. ) ;
#6391=CARTESIAN_POINT ( 'NONE',  ( 1.530808498934191521E-15, 4.250000000000000000, -25.00000000000000000 ) ) ;
#6392=LINE ( 'NONE', #5560, #2858 ) ;
#6395=LINE ( 'NONE', #5563, #10287 ) ;
#6396=AXIS2_PLACEMENT_3D ( 'NONE', #4049, #10001, #4882 ) ;
#6397=EDGE_CURVE ( 'NONE', #2342, #3364, #3863, .T. ) ;
#6399=ADVANCED_FACE ( 'NONE', ( #9980 ), #7500, .F. ) ;
#6400=ORIENTED_EDGE ( 'NONE', *, *, #9778, .F. ) ;
#6402=VERTEX_POINT ( 'NONE', #6677 ) ;
#6404=CARTESIAN_POINT ( 'NONE',  ( 17.10400172474269098, 25.00000000000000000, 12.87499999999995559 ) ) ;
#6406=DIRECTION ( 'NONE',  ( -0.8660254037844433705, 0.000000000000000000, -0.4999999999999916733 ) ) ;
#6412=VECTOR ( 'NONE', #297, 1000.000000000000000 ) ;
#6414=CIRCLE ( 'NONE', #6935, 5.999999999999999112 ) ;
#6420=VECTOR ( 'NONE', #4310, 1000.000000000000000 ) ;
#6422=CARTESIAN_POINT ( 'NONE',  ( -5.276923788646812774, -0.001000000000001000089, -15.13990010960486821 ) ) ;
#6425=ORIENTED_EDGE ( 'NONE', *, *, #9514, .T. ) ;
#6427=ORIENTED_EDGE ( 'NONE', *, *, #5640, .T. ) ;
#6431=CARTESIAN_POINT ( 'NONE',  ( -4.522825247065398226E-15, 1.143749999044084475, 24.62111388750000174 ) ) ;
#6433=CARTESIAN_POINT ( 'NONE',  ( -10.35533905932737575, 3.312500000000000000, -25.00000000000000000 ) ) ;
#6434=LINE ( 'NONE', #10676, #7919 ) ;
#6436=DIRECTION ( 'NONE',  ( 0.000000000000000000, 0.000000000000000000, 1.000000000000000000 ) ) ;
#6437=CARTESIAN_POINT ( 'NONE',  ( 25.00000000000000000, 3.612499998088169129, 0.000000000000000000 ) ) ;
#6439=VERTEX_POINT ( 'NONE', #4971 ) ;
#6441=FACE_OUTER_BOUND ( 'NONE', #2721, .T. ) ;
#6443=VERTEX_POINT ( 'NONE', #8321 ) ;
#6453=EDGE_CURVE ( 'NONE', #7963, #7140, #4913, .T. ) ;
#6454=LINE ( 'NONE', #2235, #4842 ) ;
#6455=CARTESIAN_POINT ( 'NONE',  ( 25.00000000000000000, 4.674999998088169129, -10.35533905932737753 ) ) ;
#6465=LINE ( 'NONE', #3924, #4238 ) ;
#6468=LINE ( 'NONE', #9820, #7822 ) ;
#6469=CARTESIAN_POINT ( 'NONE',  ( 24.62111388750000174, 1.218749999044084431, 0.000000000000000000 ) ) ;
#6470=ORIENTED_EDGE ( 'NONE', *, *, #8400, .T. ) ;
#6471=EDGE_CURVE ( 'NONE', #9481, #4659, #2326, .T. ) ;
#6472=VERTEX_POINT ( 'NONE', #7552 ) ;
#6475=LINE ( 'NONE', #1598, #3716 ) ;
#6476=CARTESIAN_POINT ( 'NONE',  ( 10.19839929293505953, 1.406249999044084653, -24.62111388750000174 ) ) ;
#6481=CARTESIAN_POINT ( 'NONE',  ( 0.000000000000000000, 28.00000000000000000, 0.000000000000000000 ) ) ;
#6492=CIRCLE ( 'NONE', #8070, 2.999999999999997335 ) ;
#6495=ORIENTED_EDGE ( 'NONE', *, *, #4642, .T. ) ;
#6496=( GEOMETRIC_REPRESENTATION_CONTEXT ( 3 ) GLOBAL_UNCERTAINTY_ASSIGNED_CONTEXT ( ( #10573 ) ) GLOBAL_UNIT_ASSIGNED_CONTEXT ( ( #4787, #571, #3095 ) ) REPRESENTATION_CONTEXT ( 'NONE', 'WORKASPACE' ) );
#6498=ORIENTED_EDGE ( 'NONE', *, *, #6453, .T. ) ;
#6503=CARTESIAN_POINT ( 'NONE',  ( 13.63990010960492860, 28.00000000000000000, 7.874999999999965361 ) ) ;
#6510=CARTESIAN_POINT ( 'NONE',  ( -17.40975659021753330, 3.018749999044084475, 17.40975659021752975 ) ) ;
#6514=ADVANCED_FACE ( 'NONE', ( #38 ), #10208, .F. ) ;
#6515=CARTESIAN_POINT ( 'NONE',  ( 1.530808498934191521E-15, 1.250000000000000000, -25.00000000000000000 ) ) ;
#6516=CARTESIAN_POINT ( 'NONE',  ( -17.40975659021752975, 0.5937499990440846531, -17.40975659021752975 ) ) ;
#6522=VECTOR ( 'NONE', #493, 1000.000000000000000 ) ;
#6525=CARTESIAN_POINT ( 'NONE',  ( 5.276923788646599611, 25.00000000000000000, -15.13990010960494459 ) ) ;
#6526=CARTESIAN_POINT ( 'NONE',  ( -24.62111388750000884, 3.781249999044084653, 10.19839929293505421 ) ) ;
#6527=EDGE_LOOP ( 'NONE', ( #2091, #690, #5509, #4601, #9016, #1347, #8840, #5535, #8370, #2265, #7651, #4328, #633, #10681 ) ) ;
#6532=LINE ( 'NONE', #2323, #697 ) ;
#6535=VECTOR ( 'NONE', #8338, 1000.000000000000114 ) ;
#6541=CARTESIAN_POINT ( 'NONE',  ( 1.507608415688466075E-15, 2.468749999044085097, -24.62111388750000174 ) ) ;
#6542=DIRECTION ( 'NONE',  ( -0.4999999999999887312, 0.000000000000000000, 0.8660254037844451469 ) ) ;
#6545=DIRECTION ( 'NONE',  ( 0.000000000000000000, 0.000000000000000000, 1.000000000000000000 ) ) ;
#6549=EDGE_LOOP ( 'NONE', ( #155, #2122, #7433, #9244 ) ) ;
#6554=DIRECTION ( 'NONE',  ( -0.000000000000000000, -1.000000000000000000, -0.000000000000000000 ) ) ;
#6559=PLANE ( 'NONE',  #9924 ) ;
#6560=FACE_OUTER_BOUND ( 'NONE', #901, .T. ) ;
#6562=ORIENTED_EDGE ( 'NONE', *, *, #8426, .T. ) ;
#6565=CARTESIAN_POINT ( 'NONE',  ( -17.40975659021752975, 4.768749999044084475, -17.40975659021752975 ) ) ;
#6568=CARTESIAN_POINT ( 'NONE',  ( 7.347880794884118750E-16, 28.00000000000000000, 5.999999999999999112 ) ) ;
#6571=DIRECTION ( 'NONE',  ( 0.000000000000000000, 0.000000000000000000, 1.000000000000000000 ) ) ;
#6572=CARTESIAN_POINT ( 'NONE',  ( 10.19839929293506486, 2.031249999044084653, 24.62111388749999819 ) ) ;
#6576=VERTEX_POINT ( 'NONE', #6404 ) ;
#6579=AXIS2_PLACEMENT_3D ( 'NONE', #6627, #2464, #6571 ) ;
#6581=LINE ( 'NONE', #3082, #6535 ) ;
#6583=CARTESIAN_POINT ( 'NONE',  ( 24.62111388750000174, 1.281249999044084653, -10.19839929293505776 ) ) ;
#6589=CARTESIAN_POINT ( 'NONE',  ( 19.75000000000001066, 28.00000000000000000, 2.999999999999927613 ) ) ;
#6590=AXIS2_PLACEMENT_3D ( 'NONE', #10480, #3681, #4412 ) ;
#6599=EDGE_LOOP ( 'NONE', ( #4, #10022, #7655, #5659 ) ) ;
#6602=EDGE_CURVE ( 'NONE', #5770, #7097, #2082, .T. ) ;
#6604=DIRECTION ( 'NONE',  ( 0.4999999999999951705, 0.000000000000000000, -0.8660254037844413721 ) ) ;
#6615=CARTESIAN_POINT ( 'NONE',  ( 25.00000000000000000, 4.000000000000000000, 0.000000000000000000 ) ) ;
#6620=CARTESIAN_POINT ( 'NONE',  ( -7.875000000000116351, 28.00000000000000000, -13.63990010960484334 ) ) ;
#6627=CARTESIAN_POINT ( 'NONE',  ( 0.000000000000000000, 27.99999999999999645, 0.000000000000000000 ) ) ;
#6628=CARTESIAN_POINT ( 'NONE',  ( -24.62111388750000174, 1.656249999044084431, -10.19839929293506131 ) ) ;
#6633=CARTESIAN_POINT ( 'NONE',  ( 10.19839929293506486, 3.031249999044084653, 24.62111388749999819 ) ) ;
#6634=CARTESIAN_POINT ( 'NONE',  ( 18.60400172474268032, -0.001000000000001000089, 7.276923788646641356 ) ) ;
#6635=ORIENTED_EDGE ( 'NONE', *, *, #2650, .T. ) ;
#6641=FACE_OUTER_BOUND ( 'NONE', #5527, .T. ) ;
#6645=ORIENTED_EDGE ( 'NONE', *, *, #6744, .T. ) ;
#6646=ADVANCED_FACE ( 'NONE', ( #2293 ), #9040, .F. ) ;
#6647=EDGE_CURVE ( 'NONE', #5829, #5968, #9585, .T. ) ;
#6648=CARTESIAN_POINT ( 'NONE',  ( -24.62111388750000884, 2.956249999044084475, 10.19839929293505421 ) ) ;
#6649=CARTESIAN_POINT ( 'NONE',  ( 24.62111388750000174, 0.2812499990440845976, -10.19839929293505776 ) ) ;
#6653=FACE_BOUND ( 'NONE', #6232, .T. ) ;
#6660=ORIENTED_EDGE ( 'NONE', *, *, #8877, .F. ) ;
#6661=VERTEX_POINT ( 'NONE', #4016 ) ;
#6663=ORIENTED_EDGE ( 'NONE', *, *, #2066, .T. ) ;
#6664=AXIS2_PLACEMENT_3D ( 'NONE', #6620, #3068, #4809 ) ;
#6665=VECTOR ( 'NONE', #2176, 1000.000000000000114 ) ;
#6666=LINE ( 'NONE', #10744, #8696 ) ;
#6670=CARTESIAN_POINT ( 'NONE',  ( -18.60400172474257730, 25.00000000000000000, 7.276923788646904256 ) ) ;
#6677=CARTESIAN_POINT ( 'NONE',  ( 25.00000000000000000, -2.710505431213761085E-17, 0.000000000000000000 ) ) ;
#6688=CARTESIAN_POINT ( 'NONE',  ( -24.62111388750000884, 2.781249999044085097, 10.19839929293505421 ) ) ;
#6693=ADVANCED_FACE ( 'NONE', ( #1569 ), #3158, .F. ) ;
#6694=CARTESIAN_POINT ( 'NONE',  ( 7.874999999999916511, 25.00000000000000000, -13.63990010960495702 ) ) ;
#6695=CARTESIAN_POINT ( 'NONE',  ( 24.62111388750000174, 0.2812499990440845976, -10.19839929293505776 ) ) ;
#6699=CARTESIAN_POINT ( 'NONE',  ( 17.67766952966368521, 1.487499998088169129, 17.67766952966369232 ) ) ;
#6700=DIRECTION ( 'NONE',  ( 0.000000000000000000, 1.000000000000000000, -0.000000000000000000 ) ) ;
#6704=ORIENTED_EDGE ( 'NONE', *, *, #2033, .F. ) ;
#6707=UNCERTAINTY_MEASURE_WITH_UNIT (LENGTH_MEASURE( 1.000000000000000082E-05 ), #3665, 'distance_accuracy_value', 'NONE');
#6708=CARTESIAN_POINT ( 'NONE',  ( -4.522825247065398226E-15, 2.143749999044084920, 24.62111388750000174 ) ) ;
#6710=LINE ( 'NONE', #5005, #4027 ) ;
#6716=LINE ( 'NONE', #1797, #10810 ) ;
#6717=ORIENTED_EDGE ( 'NONE', *, *, #641, .T. ) ;
#6720=AXIS2_PLACEMENT_3D ( 'NONE', #9941, #1431, #9164 ) ;
#6721=ORIENTED_EDGE ( 'NONE', *, *, #7524, .F. ) ;
#6724=CARTESIAN_POINT ( 'NONE',  ( 2.999999999999999112, 28.00000000000000000, 19.75000000000000000 ) ) ;
#6725=CARTESIAN_POINT ( 'NONE',  ( 1.285879139104720831E-15, 31.00000000000000000, 10.50000000000000000 ) ) ;
#6728=DIRECTION ( 'NONE',  ( 0.000000000000000000, -0.000000000000000000, 1.000000000000000000 ) ) ;
#6733=VERTEX_POINT ( 'NONE', #7427 ) ;
#6734=CARTESIAN_POINT ( 'NONE',  ( 17.10400172474261637, 25.00000000000000000, -9.875000000000085265 ) ) ;
#6735=VECTOR ( 'NONE', #8918, 1000.000000000000000 ) ;
#6737=ORIENTED_EDGE ( 'NONE', *, *, #106, .F. ) ;
#6738=DIRECTION ( 'NONE',  ( 1.156482317317872514E-15, 0.000000000000000000, 1.000000000000000000 ) ) ;
#6740=CARTESIAN_POINT ( 'NONE',  ( -25.00000000000000000, 5.112499998088170017, -3.061616997868383043E-15 ) ) ;
#6744=EDGE_CURVE ( 'NONE', #5745, #2067, #9971, .T. ) ;
#6747=CARTESIAN_POINT ( 'NONE',  ( 10.35533905932740240, 1.812500000000000222, 24.99999999999998224 ) ) ;
#6749=CYLINDRICAL_SURFACE ( 'NONE', #1997, 2.999999999999997335 ) ;
#6751=CARTESIAN_POINT ( 'NONE',  ( -25.00000000000001066, 1.174999998088169351, 10.35533905932737397 ) ) ;
#6756=CARTESIAN_POINT ( 'NONE',  ( 0.000000000000000000, 85.00000000000000000, 0.000000000000000000 ) ) ;
#6757=FACE_BOUND ( 'NONE', #1629, .T. ) ;
#6758=CARTESIAN_POINT ( 'NONE',  ( 1.530808498934191521E-15, 4.250000000000000000, -25.00000000000000000 ) ) ;
#6759=( BOUNDED_CURVE ( )  B_SPLINE_CURVE ( 2, ( #211, #4482, #2733, #10259, #1162, #7937, #10424, #2841, #1923 ),
 .UNSPECIFIED., .F., .F. ) 
 B_SPLINE_CURVE_WITH_KNOTS ( ( 3, 2, 2, 2, 3 ),
 ( 0.2500000000000000000, 0.2750000000000000222, 0.3000000000000000444, 0.3250000000000000666, 0.3500000000000000333 ),
 .UNSPECIFIED. ) 
 CURVE ( )  GEOMETRIC_REPRESENTATION_ITEM ( )  RATIONAL_B_SPLINE_CURVE ( ( 1.000000000000000000, 0.9238795325112867385, 1.000000000000000000, 0.9238795325112867385, 1.000000000000000000, 0.9238795325112867385, 1.000000000000000000, 0.9238795325112865164, 1.000000000000000222 ) ) 
 REPRESENTATION_ITEM ( '' )  );
#6768=CARTESIAN_POINT ( 'NONE',  ( -4.522825247065398226E-15, 1.143749999044084475, 24.62111388750000174 ) ) ;
#6769=CARTESIAN_POINT ( 'NONE',  ( 17.40975659021752975, 0.3437499990440845421, -17.40975659021752975 ) ) ;
#6773=ORIENTED_EDGE ( 'NONE', *, *, #1952, .T. ) ;
#6782=CARTESIAN_POINT ( 'NONE',  ( 12.13990010960493748, -0.001000000000001000089, 10.47307621135328759 ) ) ;
#6783=VECTOR ( 'NONE', #7372, 1000.000000000000000 ) ;
#6790=ORIENTED_EDGE ( 'NONE', *, *, #3076, .T. ) ;
#6794=DIRECTION ( 'NONE',  ( 1.000000000000000000, 0.000000000000000000, 0.000000000000000000 ) ) ;
#6799=CARTESIAN_POINT ( 'NONE',  ( -24.62111388750000884, 3.781249999044084653, 10.19839929293505421 ) ) ;
#6800=EDGE_CURVE ( 'NONE', #10642, #3303, #6666, .T. ) ;
#6801=ORIENTED_EDGE ( 'NONE', *, *, #10158, .T. ) ;
#6802=EDGE_CURVE ( 'NONE', #9220, #857, #5174, .T. ) ;
#6808=CARTESIAN_POINT ( 'NONE',  ( -7.875000000000116351, 25.00000000000000000, -13.63990010960484334 ) ) ;
#6811=DIRECTION ( 'NONE',  ( 0.5000000000000073275, -0.000000000000000000, 0.8660254037844343777 ) ) ;
#6813=ADVANCED_FACE ( 'NONE', ( #9915 ), #5830, .F. ) ;
#6815=ORIENTED_EDGE ( 'NONE', *, *, #9857, .T. ) ;
#6818=CARTESIAN_POINT ( 'NONE',  ( -2.999999999999997335, -0.001000000000001000089, 15.75000000000000355 ) ) ;
#6820=LINE ( 'NONE', #5230, #6412 ) ;
#6821=CARTESIAN_POINT ( 'NONE',  ( 17.40975659021752975, 2.518749999044084475, -17.40975659021752975 ) ) ;
#6822=CARTESIAN_POINT ( 'NONE',  ( 25.00000000000000000, 1.062500000000000222, -10.35533905932737753 ) ) ;
#6823=FILL_AREA_STYLE_COLOUR ( '', #1540 ) ;
#6826=LINE ( 'NONE', #4119, #10585 ) ;
#6830=ORIENTED_EDGE ( 'NONE', *, *, #3399, .T. ) ;
#6833=DIRECTION ( 'NONE',  ( -0.000000000000000000, -1.000000000000000000, -0.000000000000000000 ) ) ;
#6834=CARTESIAN_POINT ( 'NONE',  ( 24.62111388750000174, 0.3062499990440845643, 0.000000000000000000 ) ) ;
#6841=ORIENTED_EDGE ( 'NONE', *, *, #3837, .F. ) ;
#6848=LINE ( 'NONE', #4250, #1470 ) ;
#6850=FACE_OUTER_BOUND ( 'NONE', #1018, .T. ) ;
#6851=CARTESIAN_POINT ( 'NONE',  ( 10.19839929293506486, 5.031249999044084653, 24.62111388749999819 ) ) ;
#6858=LINE ( 'NONE', #4199, #4616 ) ;
#6859=AXIS2_PLACEMENT_3D ( 'NONE', #9272, #2532, #3598 ) ;
#6862=DIRECTION ( 'NONE',  ( 1.000000000000000000, 0.000000000000000000, -1.069128445102650095E-14 ) ) ;
#6864=FACE_BOUND ( 'NONE', #3196, .T. ) ;
#6869=ADVANCED_FACE ( 'NONE', ( #1862 ), #1038, .T. ) ;
#6871=EDGE_LOOP ( 'NONE', ( #1615, #1753, #2328, #2517, #1173 ) ) ;
#6872=EDGE_LOOP ( 'NONE', ( #966, #8923, #2257, #3480 ) ) ;
#6877=DIRECTION ( 'NONE',  ( 1.000000000000000000, 0.000000000000000000, 0.000000000000000000 ) ) ;
#6878=CARTESIAN_POINT ( 'NONE',  ( -17.67766952966369232, 3.237499998088169573, 17.67766952966368876 ) ) ;
#6879=CARTESIAN_POINT ( 'NONE',  ( 24.62111388749999463, 3.156249999044084653, 10.19839929293507730 ) ) ;
#6880=CARTESIAN_POINT ( 'NONE',  ( -10.35533905932737575, 2.924999998088169129, -25.00000000000000000 ) ) ;
#6882=FACE_BOUND ( 'NONE', #3613, .T. ) ;
#6883=DIRECTION ( 'NONE',  ( 0.000000000000000000, 0.000000000000000000, 1.000000000000000000 ) ) ;
#6885=EDGE_CURVE ( 'NONE', #3364, #3253, #40, .T. ) ;
#6888=ORIENTED_EDGE ( 'NONE', *, *, #1592, .T. ) ;
#6889=ORIENTED_EDGE ( 'NONE', *, *, #7416, .T. ) ;
#6892=ORIENTED_EDGE ( 'NONE', *, *, #9952, .T. ) ;
#6894=EDGE_CURVE ( 'NONE', #4742, #4838, #311, .T. ) ;
#6903=DIRECTION ( 'NONE',  ( -0.000000000000000000, -1.000000000000000000, -0.000000000000000000 ) ) ;
#6904=CARTESIAN_POINT ( 'NONE',  ( -17.40975659021753330, 4.018749999044084475, 17.40975659021752975 ) ) ;
#6905=AXIS2_PLACEMENT_3D ( 'NONE', #2515, #8380, #4189 ) ;
#6909=CIRCLE ( 'NONE', #5827, 25.00000000000000000 ) ;
#6912=CARTESIAN_POINT ( 'NONE',  ( -25.00000000000000000, 4.049999998088169129, -10.35533905932738108 ) ) ;
#6916=DIRECTION ( 'NONE',  ( -0.000000000000000000, -1.000000000000000000, -0.000000000000000000 ) ) ;
#6920=CARTESIAN_POINT ( 'NONE',  ( -24.62111388750000174, 4.656249999044085541, -10.19839929293506131 ) ) ;
#6922=DIRECTION ( 'NONE',  ( -0.000000000000000000, 1.000000000000000000, -0.000000000000000000 ) ) ;
#6923=CARTESIAN_POINT ( 'NONE',  ( 17.40975659021752620, 4.093749999044084653, 17.40975659021753330 ) ) ;
#6925=CARTESIAN_POINT ( 'NONE',  ( 1.507608415688466075E-15, 1.643749999044084475, -24.62111388750000174 ) ) ;
#6926=EDGE_LOOP ( 'NONE', ( #5306, #4782, #7590, #1529 ) ) ;
#6928=CARTESIAN_POINT ( 'NONE',  ( 24.99999999999999289, 1.549999998088169129, 10.35533905932739529 ) ) ;
#6931=DIRECTION ( 'NONE',  ( 0.000000000000000000, 1.000000000000000000, -0.000000000000000000 ) ) ;
#6933=AXIS2_PLACEMENT_3D ( 'NONE', #2064, #3728, #6436 ) ;
#6935=AXIS2_PLACEMENT_3D ( 'NONE', #4480, #1006, #3235 ) ;
#6936=LINE ( 'NONE', #6818, #5291 ) ;
#6939=CARTESIAN_POINT ( 'NONE',  ( -17.40975659021753330, 1.018749999044084698, 17.40975659021752975 ) ) ;
#6940=EDGE_CURVE ( 'NONE', #8379, #10642, #8161, .T. ) ;
#6941=CARTESIAN_POINT ( 'NONE',  ( -25.00000000000001421, 2.174999998088169573, 10.35533905932737397 ) ) ;
#6942=CARTESIAN_POINT ( 'NONE',  ( 24.62111388750000174, 3.218749999044084653, 0.000000000000000000 ) ) ;
#6946=CARTESIAN_POINT ( 'NONE',  ( -13.63990010960498367, 25.00000000000000000, -7.874999999999870326 ) ) ;
#6952=ORIENTED_EDGE ( 'NONE', *, *, #9343, .T. ) ;
#6954=ORIENTED_EDGE ( 'NONE', *, *, #6397, .T. ) ;
#6957=EDGE_CURVE ( 'NONE', #3898, #9950, #8714, .T. ) ;
#6958=AXIS2_PLACEMENT_3D ( 'NONE', #3925, #655, #7285 ) ;
#6963=DIRECTION ( 'NONE',  ( 0.5000000000000009992, 0.000000000000000000, 0.8660254037844380415 ) ) ;
#6967=CARTESIAN_POINT ( 'NONE',  ( 10.19839929293505953, 3.581249999044085364, -24.62111388750000174 ) ) ;
#6972=CARTESIAN_POINT ( 'NONE',  ( -4.592425496802574367E-15, 4.362499998088169129, 25.00000000000000000 ) ) ;
#6975=CARTESIAN_POINT ( 'NONE',  ( 9.875000000000023093, -0.001000000000001000089, 17.10400172474264835 ) ) ;
#6976=EDGE_CURVE ( 'NONE', #2686, #3734, #4289, .T. ) ;
#6978=DIRECTION ( 'NONE',  ( -0.000000000000000000, -1.000000000000000000, -0.000000000000000000 ) ) ;
#6979=CARTESIAN_POINT ( 'NONE',  ( -15.13990010960496235, 28.00000000000000000, -5.276923788646544544 ) ) ;
#6983=PLANE ( 'NONE',  #4603 ) ;
#6984=CARTESIAN_POINT ( 'NONE',  ( -17.67766952966369232, 2.625000000000000000, 17.67766952966368876 ) ) ;
#6985=DIRECTION ( 'NONE',  ( -1.069128445102650095E-14, 0.000000000000000000, -1.000000000000000000 ) ) ;
#6990=EDGE_CURVE ( 'NONE', #2070, #2069, #2727, .T. ) ;
#6991=CARTESIAN_POINT ( 'NONE',  ( 0.000000000000000000, 31.00000000000000000, 0.000000000000000000 ) ) ;
#6994=CARTESIAN_POINT ( 'NONE',  ( -10.35533905932737575, 4.924999998088169129, -25.00000000000000000 ) ) ;
#6995=CARTESIAN_POINT ( 'NONE',  ( 17.40975659021752620, 3.093749999044084653, 17.40975659021753330 ) ) ;
#6997=CARTESIAN_POINT ( 'NONE',  ( 13.63990010960487353, 28.00000000000000000, -4.875000000000069278 ) ) ;
#6999=CARTESIAN_POINT ( 'NONE',  ( 0.000000000000000000, 85.00000000000000000, 0.000000000000000000 ) ) ;
#7001=ORIENTED_EDGE ( 'NONE', *, *, #9628, .T. ) ;
#7003=EDGE_LOOP ( 'NONE', ( #5485, #7235 ) ) ;
#7004=ADVANCED_FACE ( 'NONE', ( #9540 ), #5352, .F. ) ;
#7005=VERTEX_POINT ( 'NONE', #9599 ) ;
#7006=DIRECTION ( 'NONE',  ( -0.000000000000000000, -1.000000000000000000, -0.000000000000000000 ) ) ;
#7009=DIRECTION ( 'NONE',  ( 0.000000000000000000, 1.000000000000000000, -0.000000000000000000 ) ) ;
#7013=DIRECTION ( 'NONE',  ( -0.000000000000000000, -1.000000000000000000, -0.000000000000000000 ) ) ;
#7019=DIRECTION ( 'NONE',  ( -0.000000000000000000, 1.000000000000000000, -0.000000000000000000 ) ) ;
#7023=CARTESIAN_POINT ( 'NONE',  ( 3.061616997868383043E-15, 85.00000000000000000, 25.00000000000000000 ) ) ;
#7024=CYLINDRICAL_SURFACE ( 'NONE', #3375, 2.999999999999997335 ) ;
#7025=CARTESIAN_POINT ( 'NONE',  ( 15.75000000000000000, 25.00000000000000000, -5.821397334365942453E-14 ) ) ;
#7027=ADVANCED_FACE ( 'NONE', ( #4933 ), #3897, .F. ) ;
#7031=CARTESIAN_POINT ( 'NONE',  ( -10.35533905932737575, 0.3125000000000000000, -25.00000000000000000 ) ) ;
#7032=CARTESIAN_POINT ( 'NONE',  ( -17.40975659021753330, 1.018749999044084698, 17.40975659021752975 ) ) ;
#7035=CARTESIAN_POINT ( 'NONE',  ( -10.35533905932739174, 2.687500000000000444, 24.99999999999999289 ) ) ;
#7039=EDGE_LOOP ( 'NONE', ( #10692, #4562, #465 ) ) ;
#7040=AXIS2_PLACEMENT_3D ( 'NONE', #1904, #3431, #7048 ) ;
#7041=VERTEX_POINT ( 'NONE', #7256 ) ;
#7042=EDGE_CURVE ( 'NONE', #2806, #2292, #8710, .T. ) ;
#7045=DIRECTION ( 'NONE',  ( 1.000000000000000000, 0.000000000000000000, -3.708321773340234242E-15 ) ) ;
#7046=CARTESIAN_POINT ( 'NONE',  ( -25.00000000000000000, 3.049999998088169129, -10.35533905932738108 ) ) ;
#7047=CARTESIAN_POINT ( 'NONE',  ( 24.99999999999999289, 4.937500000000001776, 10.35533905932739529 ) ) ;
#7048=DIRECTION ( 'NONE',  ( 1.000000000000000000, 0.000000000000000000, 0.000000000000000000 ) ) ;
#7051=PLANE ( 'NONE',  #4059 ) ;
#7052=PRODUCT_DEFINITION_CONTEXT ( 'detailed design', #1046, 'design' ) ;
#7054=DIRECTION ( 'NONE',  ( -0.000000000000000000, -1.000000000000000000, -0.000000000000000000 ) ) ;
#7055=AXIS2_PLACEMENT_3D ( 'NONE', #3426, #7695, #2593 ) ;
#7057=ORIENTED_EDGE ( 'NONE', *, *, #2747, .T. ) ;
#7058=( BOUNDED_CURVE ( )  B_SPLINE_CURVE ( 2, ( #1754, #7461, #1437, #8184, #7347, #8281, #4104, #10345, #61 ),
 .UNSPECIFIED., .F., .F. ) 
 B_SPLINE_CURVE_WITH_KNOTS ( ( 3, 2, 2, 2, 3 ),
 ( 0.2499999999999999722, 0.2750000000000000222, 0.2999999999999999889, 0.3250000000000000111, 0.3499999999999999778 ),
 .UNSPECIFIED. ) 
 CURVE ( )  GEOMETRIC_REPRESENTATION_ITEM ( )  RATIONAL_B_SPLINE_CURVE ( ( 1.000000000000000000, 0.9238795325112866275, 1.000000000000000000, 0.9238795325112867385, 1.000000000000000000, 0.9238795325112867385, 1.000000000000000000, 0.9238795325112867385, 1.000000000000000000 ) ) 
 REPRESENTATION_ITEM ( '' )  );
#7066=DIRECTION ( 'NONE',  ( -3.469446951953616950E-15, 0.000000000000000000, 1.000000000000000000 ) ) ;
#7070=VECTOR ( 'NONE', #7628, 1000.000000000000000 ) ;
#7072=CARTESIAN_POINT ( 'NONE',  ( 24.62111388750000174, 5.393749999044085364, 0.000000000000000000 ) ) ;
#7073=EDGE_CURVE ( 'NONE', #8063, #6443, #1352, .T. ) ;
#7076=DIRECTION ( 'NONE',  ( 0.000000000000000000, 1.000000000000000000, -0.000000000000000000 ) ) ;
#7077=DIRECTION ( 'NONE',  ( -0.000000000000000000, -1.000000000000000000, -0.000000000000000000 ) ) ;
#7080=CARTESIAN_POINT ( 'NONE',  ( 0.000000000000000000, 25.00000000000000000, 0.000000000000000000 ) ) ;
#7081=ADVANCED_FACE ( 'NONE', ( #9169 ), #9646, .F. ) ;
#7084=PLANE ( 'NONE',  #7581 ) ;
#7085=DIRECTION ( 'NONE',  ( -0.000000000000000000, 1.000000000000000000, -0.000000000000000000 ) ) ;
#7087=ORIENTED_EDGE ( 'NONE', *, *, #459, .T. ) ;
#7088=ADVANCED_FACE ( 'NONE', ( #2072, #8808 ), #3792, .F. ) ;
#7089=CARTESIAN_POINT ( 'NONE',  ( -3.223142256880076948E-15, -0.001000000000001000089, -15.75000000000000000 ) ) ;
#7094=AXIS2_PLACEMENT_3D ( 'NONE', #4322, #835, #2529 ) ;
#7095=ORIENTED_EDGE ( 'NONE', *, *, #8287, .F. ) ;
#7097=VERTEX_POINT ( 'NONE', #5046 ) ;
#7100=CARTESIAN_POINT ( 'NONE',  ( 10.19839929293505953, 2.581249999044084475, -24.62111388750000174 ) ) ;
#7101=CARTESIAN_POINT ( 'NONE',  ( -10.35533905932739174, 1.687500000000000000, 24.99999999999999289 ) ) ;
#7107=ORIENTED_EDGE ( 'NONE', *, *, #8080, .F. ) ;
#7109=VECTOR ( 'NONE', #1841, 1000.000000000000000 ) ;
#7110=ORIENTED_EDGE ( 'NONE', *, *, #10945, .T. ) ;
#7119=( BOUNDED_CURVE ( )  B_SPLINE_CURVE ( 2, ( #1885, #6747, #952, #230, #2003, #9562, #1942, #3646, #10389 ),
 .UNSPECIFIED., .F., .F. ) 
 B_SPLINE_CURVE_WITH_KNOTS ( ( 3, 2, 2, 2, 3 ),
 ( 0.3500000000000000333, 0.3750000000000000555, 0.4000000000000000222, 0.4249999999999999889, 0.4500000000000000111 ),
 .UNSPECIFIED. ) 
 CURVE ( )  GEOMETRIC_REPRESENTATION_ITEM ( )  RATIONAL_B_SPLINE_CURVE ( ( 0.9999999999999997780, 0.9238795325112869605, 1.000000000000000000, 0.9238795325112867385, 1.000000000000000000, 0.9238795325112867385, 1.000000000000000000, 0.9238795325112867385, 1.000000000000000000 ) ) 
 REPRESENTATION_ITEM ( '' )  );
#7121=VECTOR ( 'NONE', #980, 1000.000000000000000 ) ;
#7122=VECTOR ( 'NONE', #3228, 1000.000000000000000 ) ;
#7123=ORIENTED_EDGE ( 'NONE', *, *, #2864, .T. ) ;
#7125=DIRECTION ( 'NONE',  ( 0.000000000000000000, 0.000000000000000000, 1.000000000000000000 ) ) ;
#7126=VECTOR ( 'NONE', #927, 1000.000000000000114 ) ;
#7129=FACE_OUTER_BOUND ( 'NONE', #6872, .T. ) ;
#7131=ORIENTED_EDGE ( 'NONE', *, *, #8143, .F. ) ;
#7133=AXIS2_PLACEMENT_3D ( 'NONE', #2073, #5450, #1202 ) ;
#7139=CARTESIAN_POINT ( 'NONE',  ( 10.19839929293506486, 1.206249999044084698, 24.62111388749999819 ) ) ;
#7140=VERTEX_POINT ( 'NONE', #2531 ) ;
#7145=CARTESIAN_POINT ( 'NONE',  ( -12.47307621135344391, 28.00000000000000000, -15.60400172474256131 ) ) ;
#7147=ORIENTED_EDGE ( 'NONE', *, *, #8610, .F. ) ;
#7148=ADVANCED_FACE ( 'NONE', ( #4261 ), #4323, .F. ) ;
#7151=CARTESIAN_POINT ( 'NONE',  ( 10.19839929293505953, 1.581249999044084475, -24.62111388750000174 ) ) ;
#7152=CARTESIAN_POINT ( 'NONE',  ( 1.530808498934191521E-15, 4.250000000000000000, -25.00000000000000000 ) ) ;
#7154=FACE_OUTER_BOUND ( 'NONE', #4671, .T. ) ;
#7156=CARTESIAN_POINT ( 'NONE',  ( -10.47307621135315792, 28.00000000000000000, 12.13990010960504762 ) ) ;
#7162=DIRECTION ( 'NONE',  ( 0.000000000000000000, 1.000000000000000000, 0.000000000000000000 ) ) ;
#7163=EDGE_CURVE ( 'NONE', #5240, #8662, #7743, .T. ) ;
#7164=CARTESIAN_POINT ( 'NONE',  ( 0.000000000000000000, 0.000000000000000000, 0.000000000000000000 ) ) ;
#7166=DIRECTION ( 'NONE',  ( 1.000000000000000000, 0.000000000000000000, 0.000000000000000000 ) ) ;
#7170=EDGE_LOOP ( 'NONE', ( #5133, #5813, #8233, #3246 ) ) ;
#7174=CARTESIAN_POINT ( 'NONE',  ( 7.874999999999916511, -0.001000000000001000089, -13.63990010960495702 ) ) ;
#7176=DIRECTION ( 'NONE',  ( -0.000000000000000000, 1.000000000000000000, -0.000000000000000000 ) ) ;
#7177=CARTESIAN_POINT ( 'NONE',  ( -19.75000000000000000, 25.00000000000000000, 2.108281996628241301E-13 ) ) ;
#7182=CARTESIAN_POINT ( 'NONE',  ( 24.62111388749999108, 4.331249999044084475, 10.19839929293507730 ) ) ;
#7183=ORIENTED_EDGE ( 'NONE', *, *, #8538, .F. ) ;
#7189=ORIENTED_EDGE ( 'NONE', *, *, #7955, .F. ) ;
#7193=CARTESIAN_POINT ( 'NONE',  ( -4.522825247065398226E-15, 2.143749999044084920, 24.62111388750000174 ) ) ;
#7194=ORIENTED_EDGE ( 'NONE', *, *, #323, .F. ) ;
#7195=CARTESIAN_POINT ( 'NONE',  ( -17.67766952966369232, 1.625000000000000222, 17.67766952966368876 ) ) ;
#7198=DIRECTION ( 'NONE',  ( 0.000000000000000000, 0.000000000000000000, -1.000000000000000000 ) ) ;
#7199=CARTESIAN_POINT ( 'NONE',  ( 1.530808498934191521E-15, 0.8624999980881691286, -25.00000000000000000 ) ) ;
#7200=EDGE_CURVE ( 'NONE', #5087, #8288, #4654, .T. ) ;
#7203=AXIS2_PLACEMENT_3D ( 'NONE', #5965, #46, #10156 ) ;
#7205=EDGE_CURVE ( 'NONE', #1064, #9664, #5225, .T. ) ;
#7208=AXIS2_PLACEMENT_3D ( 'NONE', #124, #9232, #4270 ) ;
#7209=DIRECTION ( 'NONE',  ( 0.000000000000000000, 0.000000000000000000, 1.000000000000000000 ) ) ;
#7212=CARTESIAN_POINT ( 'NONE',  ( 7.276923788646575630, -0.001000000000001000089, -18.60400172474270519 ) ) ;
#7214=DIRECTION ( 'NONE',  ( 0.000000000000000000, 0.000000000000000000, 1.000000000000000000 ) ) ;
#7218=CARTESIAN_POINT ( 'NONE',  ( 3.957930336368489021E-15, -0.001000000000001000089, 22.75000000000000000 ) ) ;
#7221=CYLINDRICAL_SURFACE ( 'NONE', #9396, 5.999999999999999112 ) ;
#7222=ORIENTED_EDGE ( 'NONE', *, *, #7378, .F. ) ;
#7224=CIRCLE ( 'NONE', #2453, 20.00000000000000000 ) ;
#7225=CARTESIAN_POINT ( 'NONE',  ( 3.061616997868383043E-15, 85.00000000000000000, 25.00000000000000000 ) ) ;
#7227=CARTESIAN_POINT ( 'NONE',  ( 17.40975659021752975, 2.518749999044084475, -17.40975659021752975 ) ) ;
#7234=EDGE_CURVE ( 'NONE', #416, #5054, #10495, .T. ) ;
#7235=ORIENTED_EDGE ( 'NONE', *, *, #3491, .F. ) ;
#7236=AXIS2_PLACEMENT_3D ( 'NONE', #9306, #10370, #6963 ) ;
#7237=VERTEX_POINT ( 'NONE', #4558 ) ;
#7240=VERTEX_POINT ( 'NONE', #10395 ) ;
#7243=CARTESIAN_POINT ( 'NONE',  ( 24.62111388750000174, 1.393749999044084475, 0.000000000000000000 ) ) ;
#7244=CARTESIAN_POINT ( 'NONE',  ( 17.67766952966369232, 4.125000000000000000, -17.67766952966369232 ) ) ;
#7245=AXIS2_PLACEMENT_3D ( 'NONE', #8804, #10306, #8700 ) ;
#7247=DIRECTION ( 'NONE',  ( 1.000000000000000000, 0.000000000000000000, 0.000000000000000000 ) ) ;
#7248=DIRECTION ( 'NONE',  ( 0.000000000000000000, 0.000000000000000000, 1.000000000000000000 ) ) ;
#7249=CARTESIAN_POINT ( 'NONE',  ( 1.530808498934191521E-15, 3.250000000000000444, -25.00000000000000000 ) ) ;
#7254=LINE ( 'NONE', #2989, #1242 ) ;
#7256=CARTESIAN_POINT ( 'NONE',  ( 2.999999999999996447, 28.00000000000000000, -19.75000000000000000 ) ) ;
#7257=CARTESIAN_POINT ( 'NONE',  ( 0.000000000000000000, 85.00000000000000000, -28.00000000000000000 ) ) ;
#7259=DIRECTION ( 'NONE',  ( 0.000000000000000000, 0.000000000000000000, -1.000000000000000000 ) ) ;
#7266=ORIENTED_EDGE ( 'NONE', *, *, #1676, .T. ) ;
#7270=CARTESIAN_POINT ( 'NONE',  ( 17.67766952966368521, 4.487499998088169129, 17.67766952966369232 ) ) ;
#7272=DIRECTION ( 'NONE',  ( 0.000000000000000000, 0.000000000000000000, 1.000000000000000000 ) ) ;
#7274=AXIS2_PLACEMENT_3D ( 'NONE', #304, #9590, #8703 ) ;
#7275=VERTEX_POINT ( 'NONE', #10343 ) ;
#7281=EDGE_CURVE ( 'NONE', #2972, #7713, #5427, .T. ) ;
#7283=DIRECTION ( 'NONE',  ( -0.8660254037844407060, 0.4999999999999965583, -0.000000000000000000 ) ) ;
#7285=DIRECTION ( 'NONE',  ( 0.000000000000000000, 0.000000000000000000, 1.000000000000000000 ) ) ;
#7289=CARTESIAN_POINT ( 'NONE',  ( 24.62111388750000174, 1.281249999044084653, -10.19839929293505776 ) ) ;
#7290=VECTOR ( 'NONE', #8098, 1000.000000000000000 ) ;
#7292=VERTEX_POINT ( 'NONE', #8741 ) ;
#7296=CARTESIAN_POINT ( 'NONE',  ( -17.40975659021753330, 4.018749999044084475, 17.40975659021752975 ) ) ;
#7297=ORIENTED_EDGE ( 'NONE', *, *, #5455, .T. ) ;
#7300=CARTESIAN_POINT ( 'NONE',  ( 0.000000000000000000, 0.000000000000000000, 0.000000000000000000 ) ) ;
#7304=VERTEX_POINT ( 'NONE', #1180 ) ;
#7306=DIRECTION ( 'NONE',  ( 0.000000000000000000, 0.000000000000000000, 1.000000000000000000 ) ) ;
#7312=DIRECTION ( 'NONE',  ( -0.000000000000000000, -1.000000000000000000, -0.000000000000000000 ) ) ;
#7314=EDGE_CURVE ( 'NONE', #122, #3225, #6263, .T. ) ;
#7315=ORIENTED_EDGE ( 'NONE', *, *, #6802, .T. ) ;
#7325=EDGE_CURVE ( 'NONE', #122, #1858, #4663, .T. ) ;
#7327=DIRECTION ( 'NONE',  ( -1.000000000000000000, 0.000000000000000000, 1.069128445102650095E-14 ) ) ;
#7328=CARTESIAN_POINT ( 'NONE',  ( 18.60400172474263414, 28.00000000000000000, -7.276923788646775471 ) ) ;
#7329=CARTESIAN_POINT ( 'NONE',  ( 24.62111388750000174, 4.456249999044084475, -10.19839929293505776 ) ) ;
#7334=ORIENTED_EDGE ( 'NONE', *, *, #5735, .T. ) ;
#7337=CARTESIAN_POINT ( 'NONE',  ( 1.507608415688466075E-15, 0.4687499990440845421, -24.62111388750000174 ) ) ;
#7338=ORIENTED_EDGE ( 'NONE', *, *, #5837, .T. ) ;
#7339=ORIENTED_EDGE ( 'NONE', *, *, #2196, .T. ) ;
#7344=CARTESIAN_POINT ( 'NONE',  ( 24.62111388750000174, 3.281249999044085097, -10.19839929293505776 ) ) ;
#7345=VERTEX_POINT ( 'NONE', #10664 ) ;
#7347=CARTESIAN_POINT ( 'NONE',  ( -25.00000000000000000, 2.112499998088169129, -3.061616997868383043E-15 ) ) ;
#7349=DIRECTION ( 'NONE',  ( -0.000000000000000000, -1.000000000000000000, -0.000000000000000000 ) ) ;
#7350=DIRECTION ( 'NONE',  ( -0.000000000000000000, -1.000000000000000000, -0.000000000000000000 ) ) ;
#7356=CARTESIAN_POINT ( 'NONE',  ( 17.40975659021752975, 2.343749999044085097, -17.40975659021752975 ) ) ;
#7360=DIRECTION ( 'NONE',  ( 0.000000000000000000, 1.000000000000000000, 0.000000000000000000 ) ) ;
#7361=VECTOR ( 'NONE', #6700, 1000.000000000000000 ) ;
#7364=ORIENTED_EDGE ( 'NONE', *, *, #1952, .F. ) ;
#7366=VECTOR ( 'NONE', #9347, 1000.000000000000000 ) ;
#7368=ORIENTED_EDGE ( 'NONE', *, *, #9031, .F. ) ;
#7369=CIRCLE ( 'NONE', #5983, 2.999999999999999112 ) ;
#7372=DIRECTION ( 'NONE',  ( -0.000000000000000000, 1.000000000000000000, -0.000000000000000000 ) ) ;
#7377=( BOUNDED_CURVE ( )  B_SPLINE_CURVE ( 2, ( #10721, #7565, #8561, #5269, #5218, #9393, #3314, #4203, #5093 ),
 .UNSPECIFIED., .F., .F. ) 
 B_SPLINE_CURVE_WITH_KNOTS ( ( 3, 2, 2, 2, 3 ),
 ( 0.6500000000000000222, 0.6750000000000000444, 0.6999999999999999556, 0.7249999999999999778, 0.7500000000000000000 ),
 .UNSPECIFIED. ) 
 CURVE ( )  GEOMETRIC_REPRESENTATION_ITEM ( )  RATIONAL_B_SPLINE_CURVE ( ( 1.000000000000000000, 0.9238795325112867385, 1.000000000000000000, 0.9238795325112867385, 1.000000000000000000, 0.9238795325112867385, 1.000000000000000000, 0.9238795325112867385, 1.000000000000000000 ) ) 
 REPRESENTATION_ITEM ( '' )  );
#7378=EDGE_CURVE ( 'NONE', #3294, #2327, #3775, .T. ) ;
#7379=EDGE_CURVE ( 'NONE', #1334, #5377, #9417, .T. ) ;
#7381=CARTESIAN_POINT ( 'NONE',  ( -24.62111388750000174, 3.893749999044084475, -3.015216831376932151E-15 ) ) ;
#7386=ORIENTED_EDGE ( 'NONE', *, *, #10158, .F. ) ;
#7388=CARTESIAN_POINT ( 'NONE',  ( -4.522825247065398226E-15, 1.968749999044084653, 24.62111388750000174 ) ) ;
#7392=ORIENTED_EDGE ( 'NONE', *, *, #4234, .F. ) ;
#7394=CIRCLE ( 'NONE', #2625, 28.00000000000000000 ) ;
#7398=CARTESIAN_POINT ( 'NONE',  ( 24.62111388749999463, 1.156249999044084431, 10.19839929293507730 ) ) ;
#7400=LINE ( 'NONE', #1604, #7548 ) ;
#7401=CARTESIAN_POINT ( 'NONE',  ( 7.276923788646707969, -0.001000000000001000089, 18.60400172474265190 ) ) ;
#7410=VERTEX_POINT ( 'NONE', #6515 ) ;
#7411=ORIENTED_EDGE ( 'NONE', *, *, #1715, .T. ) ;
#7412=VECTOR ( 'NONE', #5303, 1000.000000000000114 ) ;
#7413=VECTOR ( 'NONE', #10703, 1000.000000000000000 ) ;
#7416=EDGE_CURVE ( 'NONE', #7292, #1671, #6079, .T. ) ;
#7422=CARTESIAN_POINT ( 'NONE',  ( 0.000000000000000000, 20.00000000000000355, 0.000000000000000000 ) ) ;
#7423=CIRCLE ( 'NONE', #2648, 2.999999999999997335 ) ;
#7427=CARTESIAN_POINT ( 'NONE',  ( 3.429011037612589276E-15, 0.000000000000000000, 28.00000000000000000 ) ) ;
#7429=CARTESIAN_POINT ( 'NONE',  ( -7.875000000000116351, -0.001000000000001000089, -13.63990010960484334 ) ) ;
#7431=CARTESIAN_POINT ( 'NONE',  ( 24.99999999999999289, 3.937500000000000000, 10.35533905932739529 ) ) ;
#7433=ORIENTED_EDGE ( 'NONE', *, *, #247, .F. ) ;
#7434=CIRCLE ( 'NONE', #8155, 2.999999999999999112 ) ;
#7436=ORIENTED_EDGE ( 'NONE', *, *, #3055, .F. ) ;
#7441=DIRECTION ( 'NONE',  ( 0.000000000000000000, 0.000000000000000000, 1.000000000000000000 ) ) ;
#7442=ORIENTED_EDGE ( 'NONE', *, *, #3317, .T. ) ;
#7444=CARTESIAN_POINT ( 'NONE',  ( -10.19839929293505776, 2.531249999044085097, -24.62111388750000174 ) ) ;
#7447=VERTEX_POINT ( 'NONE', #1532 ) ;
#7448=EDGE_LOOP ( 'NONE', ( #6790, #7442, #10447, #7954 ) ) ;
#7456=VECTOR ( 'NONE', #3227, 1000.000000000000000 ) ;
#7457=CARTESIAN_POINT ( 'NONE',  ( 10.19839929293505953, 2.406249999044085541, -24.62111388750000174 ) ) ;
#7460=DIRECTION ( 'NONE',  ( 0.000000000000000000, 1.000000000000000000, 0.000000000000000000 ) ) ;
#7461=CARTESIAN_POINT ( 'NONE',  ( -10.35533905932736687, 1.924999998088168907, -25.00000000000000711 ) ) ;
#7462=AXIS2_PLACEMENT_3D ( 'NONE', #147, #8478, #4233 ) ;
#7464=DIRECTION ( 'NONE',  ( 0.000000000000000000, 0.000000000000000000, 1.000000000000000000 ) ) ;
#7475=CARTESIAN_POINT ( 'NONE',  ( -17.67766952966369232, 5.237499998088169129, 17.67766952966368876 ) ) ;
#7476=CARTESIAN_POINT ( 'NONE',  ( -24.62111388750000174, 0.6562499990440846531, -10.19839929293506131 ) ) ;
#7486=EDGE_CURVE ( 'NONE', #5695, #6733, #6848, .T. ) ;
#7491=LINE ( 'NONE', #815, #4503 ) ;
#7492=DIRECTION ( 'NONE',  ( 0.8660254037844327124, 0.000000000000000000, -0.5000000000000103251 ) ) ;
#7494=EDGE_CURVE ( 'NONE', #2252, #8568, #10040, .T. ) ;
#7500=CYLINDRICAL_SURFACE ( 'NONE', #1441, 2.999999999999997335 ) ;
#7502=CARTESIAN_POINT ( 'NONE',  ( 9.875000000000023093, 28.00000000000000000, 20.10400172474264835 ) ) ;
#7506=CARTESIAN_POINT ( 'NONE',  ( -24.62111388750000884, 1.781249999044084875, 10.19839929293505421 ) ) ;
#7511=CARTESIAN_POINT ( 'NONE',  ( -24.62111388750000174, 0.7187499990440845421, -3.015216831376932151E-15 ) ) ;
#7514=ORIENTED_EDGE ( 'NONE', *, *, #508, .T. ) ;
#7516=CARTESIAN_POINT ( 'NONE',  ( -9.874999999999777955, 28.00000000000000000, 17.10400172474279401 ) ) ;
#7517=CARTESIAN_POINT ( 'NONE',  ( -7.276923788646840308, 28.00000000000000000, -18.60400172474260216 ) ) ;
#7518=LINE ( 'NONE', #7569, #556 ) ;
#7519=LINE ( 'NONE', #10898, #9335 ) ;
#7521=CARTESIAN_POINT ( 'NONE',  ( 25.00000000000000000, 5.306249999044084120, 0.000000000000000000 ) ) ;
#7523=ORIENTED_EDGE ( 'NONE', *, *, #4589, .T. ) ;
#7524=EDGE_CURVE ( 'NONE', #6576, #500, #5209, .T. ) ;
#7526=CARTESIAN_POINT ( 'NONE',  ( -17.40975659021753330, 2.018749999044084475, 17.40975659021752975 ) ) ;
#7527=CARTESIAN_POINT ( 'NONE',  ( 24.62111388750000174, 1.281249999044084653, -10.19839929293505776 ) ) ;
#7530=DIRECTION ( 'NONE',  ( 0.8660254037844433705, -0.000000000000000000, 0.4999999999999916733 ) ) ;
#7536=EDGE_LOOP ( 'NONE', ( #8170, #8177, #7868, #6062 ) ) ;
#7537=ORIENTED_EDGE ( 'NONE', *, *, #398, .F. ) ;
#7544=CARTESIAN_POINT ( 'NONE',  ( -13.63990010960498367, -0.001000000000001000089, -4.874999999999872102 ) ) ;
#7546=EDGE_CURVE ( 'NONE', #3125, #7292, #10882, .T. ) ;
#7547=AXIS2_PLACEMENT_3D ( 'NONE', #1190, #7877, #4571 ) ;
#7548=VECTOR ( 'NONE', #2322, 1000.000000000000000 ) ;
#7552=CARTESIAN_POINT ( 'NONE',  ( -4.592425496802574367E-15, 0.7500000000000000000, 25.00000000000000000 ) ) ;
#7556=CARTESIAN_POINT ( 'NONE',  ( -15.13990010960484867, 25.00000000000000000, 5.276923788646865177 ) ) ;
#7557=VERTEX_POINT ( 'NONE', #7556 ) ;
#7559=CARTESIAN_POINT ( 'NONE',  ( -17.40975659021753330, 3.843749999044085097, 17.40975659021752975 ) ) ;
#7562=CARTESIAN_POINT ( 'NONE',  ( -10.19839929293507552, 0.9062499990440844311, 24.62111388749999463 ) ) ;
#7563=CARTESIAN_POINT ( 'NONE',  ( -12.47307621135344391, 25.00000000000000000, -15.60400172474256131 ) ) ;
#7564=ORIENTED_EDGE ( 'NONE', *, *, #7073, .F. ) ;
#7565=CARTESIAN_POINT ( 'NONE',  ( -10.35533905932737575, 3.312500000000000000, -25.00000000000000000 ) ) ;
#7568=DIRECTION ( 'NONE',  ( 0.000000000000000000, 0.000000000000000000, 1.000000000000000000 ) ) ;
#7569=CARTESIAN_POINT ( 'NONE',  ( 18.60400172474268032, -0.001000000000001000089, 7.276923788646641356 ) ) ;
#7570=CARTESIAN_POINT ( 'NONE',  ( 10.47307621135332667, 25.00000000000000000, 12.13990010960489840 ) ) ;
#7574=EDGE_LOOP ( 'NONE', ( #6815, #3810, #6269, #7621 ) ) ;
#7575=ORIENTED_EDGE ( 'NONE', *, *, #436, .F. ) ;
#7577=CARTESIAN_POINT ( 'NONE',  ( -10.19839929293507552, 1.081249999044084475, 24.62111388749999463 ) ) ;
#7578=CARTESIAN_POINT ( 'NONE',  ( 24.62111388750000174, 2.281249999044085541, -10.19839929293505776 ) ) ;
#7581=AXIS2_PLACEMENT_3D ( 'NONE', #7858, #8052, #6302 ) ;
#7587=ORIENTED_EDGE ( 'NONE', *, *, #5211, .F. ) ;
#7589=ORIENTED_EDGE ( 'NONE', *, *, #5704, .T. ) ;
#7590=ORIENTED_EDGE ( 'NONE', *, *, #9075, .T. ) ;
#7592=CIRCLE ( 'NONE', #2824, 25.00000000000000000 ) ;
#7596=PLANE ( 'NONE',  #5016 ) ;
#7597=LINE ( 'NONE', #864, #10486 ) ;
#7601=ORIENTED_EDGE ( 'NONE', *, *, #7846, .F. ) ;
#7613=ORIENTED_EDGE ( 'NONE', *, *, #1144, .T. ) ;
#7620=CARTESIAN_POINT ( 'NONE',  ( 0.000000000000000000, 85.00000000000000000, 0.000000000000000000 ) ) ;
#7621=ORIENTED_EDGE ( 'NONE', *, *, #10512, .F. ) ;
#7622=CARTESIAN_POINT ( 'NONE',  ( 12.47307621135333200, -0.001000000000001000089, 15.60400172474264835 ) ) ;
#7624=DIRECTION ( 'NONE',  ( -0.000000000000000000, 1.000000000000000000, -0.000000000000000000 ) ) ;
#7628=DIRECTION ( 'NONE',  ( -0.000000000000000000, -1.000000000000000000, -0.000000000000000000 ) ) ;
#7634=ORIENTED_EDGE ( 'NONE', *, *, #1075, .T. ) ;
#7638=CARTESIAN_POINT ( 'NONE',  ( 17.40975659021752620, 2.268749999044084475, 17.40975659021753330 ) ) ;
#7640=CARTESIAN_POINT ( 'NONE',  ( -24.62111388750000174, 3.718749999044084653, -3.015216831376932151E-15 ) ) ;
#7648=ORIENTED_EDGE ( 'NONE', *, *, #3755, .F. ) ;
#7649=EDGE_LOOP ( 'NONE', ( #6888, #8272, #5116 ) ) ;
#7651=ORIENTED_EDGE ( 'NONE', *, *, #5590, .T. ) ;
#7655=ORIENTED_EDGE ( 'NONE', *, *, #4796, .T. ) ;
#7656=EDGE_CURVE ( 'NONE', #500, #10484, #1641, .T. ) ;
#7659=DIRECTION ( 'NONE',  ( 0.5000000000000073275, 0.000000000000000000, 0.8660254037844343777 ) ) ;
#7664=ORIENTED_EDGE ( 'NONE', *, *, #9778, .T. ) ;
#7665=CARTESIAN_POINT ( 'NONE',  ( -4.592425496802574367E-15, 4.750000000000000000, 25.00000000000000000 ) ) ;
#7667=CARTESIAN_POINT ( 'NONE',  ( 10.35533905932742016, 5.424999998088169129, 24.99999999999996447 ) ) ;
#7670=EDGE_CURVE ( 'NONE', #3699, #716, #3393, .T. ) ;
#7675=CARTESIAN_POINT ( 'NONE',  ( -24.62111388750000174, 3.656249999044084653, -10.19839929293506131 ) ) ;
#7676=ADVANCED_FACE ( 'NONE', ( #1995 ), #5460, .F. ) ;
#7688=CARTESIAN_POINT ( 'NONE',  ( -7.276923788646840308, 25.00000000000000000, -18.60400172474260216 ) ) ;
#7691=ORIENTED_EDGE ( 'NONE', *, *, #2012, .T. ) ;
#7693=ORIENTED_EDGE ( 'NONE', *, *, #792, .F. ) ;
#7695=DIRECTION ( 'NONE',  ( 1.000000000000000000, 0.000000000000000000, -2.168404344971010347E-16 ) ) ;
#7697=CARTESIAN_POINT ( 'NONE',  ( -24.62111388750000174, 0.8312499990440845865, -10.19839929293506131 ) ) ;
#7698=CARTESIAN_POINT ( 'NONE',  ( -17.40975659021752975, 2.768749999044084475, -17.40975659021752975 ) ) ;
#7699=CARTESIAN_POINT ( 'NONE',  ( -4.522825247065398226E-15, 4.968749999044083765, 24.62111388750000174 ) ) ;
#7702=FACE_BOUND ( 'NONE', #1783, .T. ) ;
#7703=DIRECTION ( 'NONE',  ( -0.000000000000000000, -1.000000000000000000, -0.000000000000000000 ) ) ;
#7705=ORIENTED_EDGE ( 'NONE', *, *, #2807, .F. ) ;
#7708=ORIENTED_EDGE ( 'NONE', *, *, #8885, .T. ) ;
#7709=EDGE_LOOP ( 'NONE', ( #9083, #10902, #8531, #10346, #902 ) ) ;
#7710=CARTESIAN_POINT ( 'NONE',  ( 18.60400172474263414, -0.001000000000001000089, -7.276923788646775471 ) ) ;
#7713=VERTEX_POINT ( 'NONE', #4548 ) ;
#7718=DIRECTION ( 'NONE',  ( 0.000000000000000000, 0.000000000000000000, 1.000000000000000000 ) ) ;
#7720=VECTOR ( 'NONE', #1991, 1000.000000000000000 ) ;
#7727=DIRECTION ( 'NONE',  ( 0.8660254037844399289, 0.000000000000000000, 0.4999999999999978351 ) ) ;
#7728=STYLED_ITEM ( 'NONE', ( #2163 ), #715 ) ;
#7729=CARTESIAN_POINT ( 'NONE',  ( 0.000000000000000000, 85.00000000000000000, 0.000000000000000000 ) ) ;
#7731=AXIS2_PLACEMENT_3D ( 'NONE', #4772, #2109, #10619 ) ;
#7736=LINE ( 'NONE', #2471, #534 ) ;
#7738=CARTESIAN_POINT ( 'NONE',  ( -17.40975659021753330, 4.843749999044083765, 17.40975659021752975 ) ) ;
#7739=CARTESIAN_POINT ( 'NONE',  ( 10.19839929293505953, 1.581249999044084475, -24.62111388750000174 ) ) ;
#7741=CARTESIAN_POINT ( 'NONE',  ( -10.35533905932739174, 1.299999998088168907, 24.99999999999999289 ) ) ;
#7743=LINE ( 'NONE', #2579, #2345 ) ;
#7744=CARTESIAN_POINT ( 'NONE',  ( 7.276923788646576519, 25.00000000000000000, -18.60400172474270519 ) ) ;
#7753=CARTESIAN_POINT ( 'NONE',  ( -24.62111388750000884, 0.9562499990440846975, 10.19839929293505421 ) ) ;
#7754=CARTESIAN_POINT ( 'NONE',  ( 25.00000000000000000, 4.674999998088169129, -10.35533905932737753 ) ) ;
#7755=CARTESIAN_POINT ( 'NONE',  ( 24.62111388750000174, 3.281249999044085097, -10.19839929293505776 ) ) ;
#7756=CARTESIAN_POINT ( 'NONE',  ( -10.35533905932739174, 3.299999998088169129, 24.99999999999999289 ) ) ;
#7767=VERTEX_POINT ( 'NONE', #6298 ) ;
#7772=VECTOR ( 'NONE', #4048, 1000.000000000000000 ) ;
#7773=ADVANCED_FACE ( 'NONE', ( #3584 ), #6136, .F. ) ;
#7774=CARTESIAN_POINT ( 'NONE',  ( -10.47307621135341904, -0.001000000000001000089, -12.13990010960482557 ) ) ;
#7779=CARTESIAN_POINT ( 'NONE',  ( -15.13990010960496235, -0.001000000000001000089, -5.276923788646544544 ) ) ;
#7781=VECTOR ( 'NONE', #3458, 999.9999999999998863 ) ;
#7783=ORIENTED_EDGE ( 'NONE', *, *, #6453, .F. ) ;
#7790=SHAPE_DEFINITION_REPRESENTATION ( #9332, #5021 ) ;
#7792=DIRECTION ( 'NONE',  ( 0.000000000000000000, -0.000000000000000000, 1.000000000000000000 ) ) ;
#7794=ORIENTED_EDGE ( 'NONE', *, *, #7314, .F. ) ;
#7801=CARTESIAN_POINT ( 'NONE',  ( -17.67766952966369232, 1.237499998088169129, 17.67766952966368876 ) ) ;
#7806=AXIS2_PLACEMENT_3D ( 'NONE', #9735, #5550, #7464 ) ;
#7807=ORIENTED_EDGE ( 'NONE', *, *, #8198, .T. ) ;
#7815=CARTESIAN_POINT ( 'NONE',  ( -17.67766952966368876, 2.987499998088169129, -17.67766952966369232 ) ) ;
#7816=CARTESIAN_POINT ( 'NONE',  ( -10.19839929293507552, 4.906249999044083765, 24.62111388749999463 ) ) ;
#7817=CARTESIAN_POINT ( 'NONE',  ( 1.530808498934191521E-15, 2.862499998088169573, -25.00000000000000000 ) ) ;
#7818=ADVANCED_FACE ( 'NONE', ( #4427 ), #7024, .F. ) ;
#7820=CARTESIAN_POINT ( 'NONE',  ( 0.000000000000000000, 25.00000000000000000, 0.000000000000000000 ) ) ;
#7821=CARTESIAN_POINT ( 'NONE',  ( 0.000000000000000000, 85.00000000000000000, -25.00000000000000000 ) ) ;
#7822=VECTOR ( 'NONE', #2254, 1000.000000000000000 ) ;
#7830=VERTEX_POINT ( 'NONE', #6349 ) ;
#7831=AXIS2_PLACEMENT_3D ( 'NONE', #7164, #1250, #4689 ) ;
#7832=FACE_OUTER_BOUND ( 'NONE', #2103, .T. ) ;
#7835=DIRECTION ( 'NONE',  ( -0.000000000000000000, 1.000000000000000000, -0.000000000000000000 ) ) ;
#7837=DIRECTION ( 'NONE',  ( 0.000000000000000000, 0.000000000000000000, 1.000000000000000000 ) ) ;
#7839=CARTESIAN_POINT ( 'NONE',  ( -17.10400172474254532, -0.001000000000001000089, 9.875000000000202505 ) ) ;
#7842=CARTESIAN_POINT ( 'NONE',  ( -7.875000000000116351, 28.00000000000000000, -10.63990010960484334 ) ) ;
#7843=EDGE_CURVE ( 'NONE', #3931, #10673, #2295, .T. ) ;
#7844=ORIENTED_EDGE ( 'NONE', *, *, #6280, .T. ) ;
#7846=EDGE_CURVE ( 'NONE', #5377, #1334, #1651, .T. ) ;
#7849=CYLINDRICAL_SURFACE ( 'NONE', #4629, 2.999999999999997335 ) ;
#7850=LINE ( 'NONE', #1931, #7720 ) ;
#7855=DIRECTION ( 'NONE',  ( -0.000000000000000000, -1.000000000000000000, -0.000000000000000000 ) ) ;
#7858=CARTESIAN_POINT ( 'NONE',  ( -2.999999999999996447, -0.001000000000001000089, 19.75000000000000000 ) ) ;
#7860=CARTESIAN_POINT ( 'NONE',  ( 24.62111388750000174, 0.4562499990440845310, -10.19839929293505776 ) ) ;
#7865=FACE_BOUND ( 'NONE', #582, .T. ) ;
#7868=ORIENTED_EDGE ( 'NONE', *, *, #2932, .T. ) ;
#7870=ORIENTED_EDGE ( 'NONE', *, *, #1732, .T. ) ;
#7872=CARTESIAN_POINT ( 'NONE',  ( -2.999999999999999112, 25.00000000000000000, -19.75000000000000000 ) ) ;
#7875=CARTESIAN_POINT ( 'NONE',  ( 17.67766952966368521, 2.487499998088169129, 17.67766952966369232 ) ) ;
#7876=CARTESIAN_POINT ( 'NONE',  ( 1.530808498934191521E-15, 0.2500000000000000000, -25.00000000000000000 ) ) ;
#7877=DIRECTION ( 'NONE',  ( -0.000000000000000000, 1.000000000000000000, 0.000000000000000000 ) ) ;
#7879=CARTESIAN_POINT ( 'NONE',  ( -5.276923788646491253, 28.00000000000000000, 15.13990010960497834 ) ) ;
#7885=EDGE_CURVE ( 'NONE', #7767, #1673, #1479, .T. ) ;
#7888=DIRECTION ( 'NONE',  ( 0.000000000000000000, 0.000000000000000000, -1.000000000000000000 ) ) ;
#7889=CARTESIAN_POINT ( 'NONE',  ( 0.000000000000000000, 85.00000000000000000, 0.000000000000000000 ) ) ;
#7891=LINE ( 'NONE', #368, #64 ) ;
#7895=CARTESIAN_POINT ( 'NONE',  ( 24.62111388749999463, 5.331249999044085364, 10.19839929293507730 ) ) ;
#7899=VERTEX_POINT ( 'NONE', #9042 ) ;
#7900=EDGE_CURVE ( 'NONE', #2289, #6733, #5355, .T. ) ;
#7901=SURFACE_SIDE_STYLE ('',( #2846 ) ) ;
#7906=CARTESIAN_POINT ( 'NONE',  ( 3.429011037612589276E-15, 85.00000000000000000, 28.00000000000000000 ) ) ;
#7909=CARTESIAN_POINT ( 'NONE',  ( 2.999999999999999112, 25.00000000000000000, 19.75000000000000000 ) ) ;
#7910=AXIS2_PLACEMENT_3D ( 'NONE', #10546, #7085, #4705 ) ;
#7912=LINE ( 'NONE', #2805, #5507 ) ;
#7917=CARTESIAN_POINT ( 'NONE',  ( -4.592425496802574367E-15, 2.362499998088169129, 25.00000000000000000 ) ) ;
#7918=ORIENTED_EDGE ( 'NONE', *, *, #3552, .F. ) ;
#7919=VECTOR ( 'NONE', #3086, 1000.000000000000114 ) ;
#7922=CARTESIAN_POINT ( 'NONE',  ( -24.62111388750000174, 4.831249999044085364, -10.19839929293506131 ) ) ;
#7923=CARTESIAN_POINT ( 'NONE',  ( 17.67766952966368521, 3.875000000000000000, 17.67766952966369232 ) ) ;
#7925=DIRECTION ( 'NONE',  ( -2.168404344971010347E-16, 0.000000000000000000, -1.000000000000000000 ) ) ;
#7929=CIRCLE ( 'NONE', #9510, 10.50000000000000000 ) ;
#7930=ORIENTED_EDGE ( 'NONE', *, *, #5704, .F. ) ;
#7932=DIRECTION ( 'NONE',  ( -0.5000000000000073275, 0.000000000000000000, -0.8660254037844344888 ) ) ;
#7937=CARTESIAN_POINT ( 'NONE',  ( -25.00000000000001066, 1.562500000000000000, 10.35533905932737397 ) ) ;
#7938=CARTESIAN_POINT ( 'NONE',  ( 24.62111388750000174, 4.393749999044084475, 0.000000000000000000 ) ) ;
#7939=VERTEX_POINT ( 'NONE', #640 ) ;
#7940=AXIS2_PLACEMENT_3D ( 'NONE', #7622, #1889, #3354 ) ;
#7951=ADVANCED_FACE ( 'NONE', ( #3160 ), #8983, .F. ) ;
#7954=ORIENTED_EDGE ( 'NONE', *, *, #6397, .F. ) ;
#7955=EDGE_CURVE ( 'NONE', #9592, #5068, #1052, .T. ) ;
#7958=VECTOR ( 'NONE', #8209, 1000.000000000000000 ) ;
#7963=VERTEX_POINT ( 'NONE', #5024 ) ;
#7968=CARTESIAN_POINT ( 'NONE',  ( 24.99999999999999289, 2.549999998088169129, 10.35533905932739529 ) ) ;
#7970=VERTEX_POINT ( 'NONE', #3446 ) ;
#7971=EDGE_CURVE ( 'NONE', #2327, #7970, #7597, .T. ) ;
#7974=CARTESIAN_POINT ( 'NONE',  ( 10.19839929293506486, 2.206249999044084920, 24.62111388749999819 ) ) ;
#7975=CARTESIAN_POINT ( 'NONE',  ( -17.67766952966368876, 4.375000000000000000, -17.67766952966369232 ) ) ;
#7978=CARTESIAN_POINT ( 'NONE',  ( 24.81055694375000087, 5.503124998566127246, 0.000000000000000000 ) ) ;
#7988=AXIS2_PLACEMENT_3D ( 'NONE', #1204, #3682, #264 ) ;
#7991=DIRECTION ( 'NONE',  ( 0.000000000000000000, 0.000000000000000000, 1.000000000000000000 ) ) ;
#7992=CARTESIAN_POINT ( 'NONE',  ( 2.999999999999999112, 28.00000000000000000, 19.75000000000000000 ) ) ;
#7993=EDGE_LOOP ( 'NONE', ( #5658, #7334, #6717, #562 ) ) ;
#7995=ORIENTED_EDGE ( 'NONE', *, *, #2321, .T. ) ;
#8001=CYLINDRICAL_SURFACE ( 'NONE', #10648, 25.00000000000000000 ) ;
#8004=CARTESIAN_POINT ( 'NONE',  ( 9.875000000000023093, -0.001000000000001000089, 20.10400172474264835 ) ) ;
#8007=ORIENTED_EDGE ( 'NONE', *, *, #1960, .T. ) ;
#8013=CARTESIAN_POINT ( 'NONE',  ( 10.19839929293505953, 2.581249999044084920, -24.62111388750000174 ) ) ;
#8016=CARTESIAN_POINT ( 'NONE',  ( -4.592425496802574367E-15, 2.750000000000000000, 25.00000000000000000 ) ) ;
#8021=ORIENTED_EDGE ( 'NONE', *, *, #1676, .F. ) ;
#8025=CARTESIAN_POINT ( 'NONE',  ( -24.62111388750000884, 4.956249999044084475, 10.19839929293505421 ) ) ;
#8027=CARTESIAN_POINT ( 'NONE',  ( -10.35533905932737575, 2.312500000000000888, -25.00000000000000000 ) ) ;
#8029=CARTESIAN_POINT ( 'NONE',  ( 17.67766952966369232, 1.737499998088169351, -17.67766952966369232 ) ) ;
#8032=CARTESIAN_POINT ( 'NONE',  ( 10.35533905932739174, 0.8125000000000001110, 24.99999999999998934 ) ) ;
#8033=ADVANCED_FACE ( 'NONE', ( #755 ), #3387, .F. ) ;
#8034=ORIENTED_EDGE ( 'NONE', *, *, #3331, .F. ) ;
#8035=ORIENTED_EDGE ( 'NONE', *, *, #9372, .T. ) ;
#8036=ORIENTED_EDGE ( 'NONE', *, *, #9560, .T. ) ;
#8040=CARTESIAN_POINT ( 'NONE',  ( -15.75000000000000000, -0.001000000000001000089, 1.681956355172181189E-13 ) ) ;
#8042=( BOUNDED_CURVE ( )  B_SPLINE_CURVE ( 2, ( #3398, #993, #4359, #6912, #3517, #3336, #5029, #216, #6972 ),
 .UNSPECIFIED., .F., .F. ) 
 B_SPLINE_CURVE_WITH_KNOTS ( ( 3, 2, 2, 2, 3 ),
 ( 0.6500000000000000222, 0.6750000000000000444, 0.6999999999999999556, 0.7249999999999999778, 0.7500000000000000000 ),
 .UNSPECIFIED. ) 
 CURVE ( )  GEOMETRIC_REPRESENTATION_ITEM ( )  RATIONAL_B_SPLINE_CURVE ( ( 1.000000000000000000, 0.9238795325112867385, 1.000000000000000000, 0.9238795325112867385, 1.000000000000000000, 0.9238795325112867385, 1.000000000000000000, 0.9238795325112867385, 1.000000000000000000 ) ) 
 REPRESENTATION_ITEM ( '' )  );
#8043=CARTESIAN_POINT ( 'NONE',  ( 3.223142256880076948E-15, -0.001000000000001000089, 15.75000000000000000 ) ) ;
#8044=ORIENTED_EDGE ( 'NONE', *, *, #1331, .F. ) ;
#8051=ORIENTED_EDGE ( 'NONE', *, *, #9514, .F. ) ;
#8052=DIRECTION ( 'NONE',  ( -1.000000000000000000, 0.000000000000000000, 2.168404344971010347E-16 ) ) ;
#8054=CARTESIAN_POINT ( 'NONE',  ( 24.62111388750000174, 5.393749999044085364, 0.000000000000000000 ) ) ;
#8063=VERTEX_POINT ( 'NONE', #5125 ) ;
#8070=AXIS2_PLACEMENT_3D ( 'NONE', #8475, #6833, #6003 ) ;
#8071=CARTESIAN_POINT ( 'NONE',  ( -17.40975659021752975, 3.768749999044084475, -17.40975659021752975 ) ) ;
#8073=CARTESIAN_POINT ( 'NONE',  ( 25.00000000000000000, 4.000000000000000000, 0.000000000000000000 ) ) ;
#8077=DIRECTION ( 'NONE',  ( 0.000000000000000000, 1.000000000000000000, 0.000000000000000000 ) ) ;
#8078=CARTESIAN_POINT ( 'NONE',  ( 24.99999999999999289, 3.549999998088169573, 10.35533905932739529 ) ) ;
#8080=EDGE_CURVE ( 'NONE', #1429, #10131, #7491, .T. ) ;
#8091=DIRECTION ( 'NONE',  ( 0.000000000000000000, 1.000000000000000000, 0.000000000000000000 ) ) ;
#8092=CARTESIAN_POINT ( 'NONE',  ( 3.061616997868383043E-15, 85.00000000000000000, 25.00000000000000000 ) ) ;
#8095=ORIENTED_EDGE ( 'NONE', *, *, #7670, .F. ) ;
#8098=DIRECTION ( 'NONE',  ( -0.000000000000000000, 1.000000000000000000, -0.000000000000000000 ) ) ;
#8099=CARTESIAN_POINT ( 'NONE',  ( 0.000000000000000000, 0.000000000000000000, 0.000000000000000000 ) ) ;
#8101=DIRECTION ( 'NONE',  ( -0.000000000000000000, -1.000000000000000000, -0.000000000000000000 ) ) ;
#8104=VERTEX_POINT ( 'NONE', #10925 ) ;
#8109=CARTESIAN_POINT ( 'NONE',  ( 24.62111388750000174, 2.393749999044084475, 0.000000000000000000 ) ) ;
#8110=ORIENTED_EDGE ( 'NONE', *, *, #3823, .T. ) ;
#8117=VECTOR ( 'NONE', #928, 1000.000000000000000 ) ;
#8118=VERTEX_POINT ( 'NONE', #6725 ) ;
#8120=ORIENTED_EDGE ( 'NONE', *, *, #10324, .T. ) ;
#8123=CARTESIAN_POINT ( 'NONE',  ( -24.62111388750000174, 2.831249999044084475, -10.19839929293506131 ) ) ;
#8126=CARTESIAN_POINT ( 'NONE',  ( 17.67766952966368521, 1.875000000000000000, 17.67766952966369232 ) ) ;
#8127=AXIS2_PLACEMENT_3D ( 'NONE', #4401, #4575, #1193 ) ;
#8129=CYLINDRICAL_SURFACE ( 'NONE', #2946, 28.00000000000000000 ) ;
#8132=CARTESIAN_POINT ( 'NONE',  ( 17.67766952966368521, 0.8750000000000000000, 17.67766952966369232 ) ) ;
#8143=EDGE_CURVE ( 'NONE', #10668, #4321, #7891, .T. ) ;
#8153=EDGE_CURVE ( 'NONE', #4266, #6402, #4650, .T. ) ;
#8155=AXIS2_PLACEMENT_3D ( 'NONE', #4749, #5734, #7272 ) ;
#8159=CARTESIAN_POINT ( 'NONE',  ( 17.67766952966369232, 0.1249999999999999722, -17.67766952966369232 ) ) ;
#8160=DIRECTION ( 'NONE',  ( -0.000000000000000000, 1.000000000000000000, -0.000000000000000000 ) ) ;
#8161=CIRCLE ( 'NONE', #10628, 2.999999999999998668 ) ;
#8166=AXIS2_PLACEMENT_3D ( 'NONE', #7025, #7855, #4550 ) ;
#8169=CARTESIAN_POINT ( 'NONE',  ( -17.40975659021752975, 3.768749999044084475, -17.40975659021752975 ) ) ;
#8170=ORIENTED_EDGE ( 'NONE', *, *, #7314, .T. ) ;
#8177=ORIENTED_EDGE ( 'NONE', *, *, #66, .T. ) ;
#8179=AXIS2_PLACEMENT_3D ( 'NONE', #2043, #2850, #1217 ) ;
#8182=CARTESIAN_POINT ( 'NONE',  ( 24.62111388749999463, 2.156249999044085097, 10.19839929293507730 ) ) ;
#8183=ORIENTED_EDGE ( 'NONE', *, *, #10512, .T. ) ;
#8184=CARTESIAN_POINT ( 'NONE',  ( -25.00000000000000000, 2.049999998088169129, -10.35533905932738108 ) ) ;
#8189=VERTEX_POINT ( 'NONE', #983 ) ;
#8190=ORIENTED_EDGE ( 'NONE', *, *, #6268, .F. ) ;
#8191=CARTESIAN_POINT ( 'NONE',  ( 1.507608415688466075E-15, 1.468749999044084431, -24.62111388750000174 ) ) ;
#8198=EDGE_CURVE ( 'NONE', #6576, #122, #1815, .T. ) ;
#8200=EDGE_CURVE ( 'NONE', #7140, #6576, #933, .T. ) ;
#8201=CARTESIAN_POINT ( 'NONE',  ( -13.63990010960498367, 25.00000000000000000, -7.874999999999870326 ) ) ;
#8204=DIRECTION ( 'NONE',  ( -0.000000000000000000, 1.000000000000000000, -0.000000000000000000 ) ) ;
#8205=ADVANCED_FACE ( 'NONE', ( #1920 ), #9543, .F. ) ;
#8206=ORIENTED_EDGE ( 'NONE', *, *, #7846, .T. ) ;
#8209=DIRECTION ( 'NONE',  ( 0.000000000000000000, 1.000000000000000000, -0.000000000000000000 ) ) ;
#8210=CARTESIAN_POINT ( 'NONE',  ( 17.40975659021752620, 3.268749999044084475, 17.40975659021753330 ) ) ;
#8211=ORIENTED_EDGE ( 'NONE', *, *, #8685, .F. ) ;
#8212=DIRECTION ( 'NONE',  ( 0.8660254037844361541, 0.000000000000000000, -0.5000000000000042188 ) ) ;
#8217=CARTESIAN_POINT ( 'NONE',  ( 10.19839929293505953, 1.406249999044084209, -24.62111388750000174 ) ) ;
#8218=ORIENTED_EDGE ( 'NONE', *, *, #4721, .F. ) ;
#8225=CARTESIAN_POINT ( 'NONE',  ( 1.507608415688466075E-15, 0.4687499990440845421, -24.62111388750000174 ) ) ;
#8227=DIRECTION ( 'NONE',  ( -0.000000000000000000, 1.000000000000000000, -0.000000000000000000 ) ) ;
#8232=ORIENTED_EDGE ( 'NONE', *, *, #9839, .T. ) ;
#8233=ORIENTED_EDGE ( 'NONE', *, *, #10640, .F. ) ;
#8234=ORIENTED_EDGE ( 'NONE', *, *, #5144, .F. ) ;
#8237=CARTESIAN_POINT ( 'NONE',  ( -10.19839929293505776, 2.531249999044085097, -24.62111388750000174 ) ) ;
#8239=AXIS2_PLACEMENT_3D ( 'NONE', #1875, #10091, #2562 ) ;
#8241=DIRECTION ( 'NONE',  ( 2.312964634635745028E-15, 0.000000000000000000, 1.000000000000000000 ) ) ;
#8245=EDGE_LOOP ( 'NONE', ( #3558, #9678, #6892, #321 ) ) ;
#8249=ORIENTED_EDGE ( 'NONE', *, *, #323, .T. ) ;
#8252=ADVANCED_FACE ( 'NONE', ( #1099 ), #9601, .F. ) ;
#8255=CARTESIAN_POINT ( 'NONE',  ( -4.592425496802574367E-15, 2.362499998088169129, 25.00000000000000000 ) ) ;
#8266=ORIENTED_EDGE ( 'NONE', *, *, #3817, .T. ) ;
#8268=CARTESIAN_POINT ( 'NONE',  ( 17.40975659021752620, 1.093749999044084653, 17.40975659021753330 ) ) ;
#8271=EDGE_LOOP ( 'NONE', ( #4406, #5673, #6660, #621 ) ) ;
#8272=ORIENTED_EDGE ( 'NONE', *, *, #2807, .T. ) ;
#8273=AXIS2_PLACEMENT_3D ( 'NONE', #4154, #10779, #10893 ) ;
#8277=CARTESIAN_POINT ( 'NONE',  ( 1.507608415688466075E-15, 3.468749999044085097, -24.62111388750000174 ) ) ;
#8279=FACE_OUTER_BOUND ( 'NONE', #3513, .T. ) ;
#8281=CARTESIAN_POINT ( 'NONE',  ( -25.00000000000001066, 2.174999998088168685, 10.35533905932737397 ) ) ;
#8283=DIRECTION ( 'NONE',  ( 0.000000000000000000, -0.000000000000000000, 1.000000000000000000 ) ) ;
#8285=VECTOR ( 'NONE', #10382, 1000.000000000000000 ) ;
#8287=EDGE_CURVE ( 'NONE', #9951, #120, #402, .T. ) ;
#8288=VERTEX_POINT ( 'NONE', #10689 ) ;
#8289=ORIENTED_EDGE ( 'NONE', *, *, #119, .F. ) ;
#8294=CARTESIAN_POINT ( 'NONE',  ( -24.62111388750000884, 0.9562499990440846975, 10.19839929293505421 ) ) ;
#8295=DIRECTION ( 'NONE',  ( -0.000000000000000000, 1.000000000000000000, -0.000000000000000000 ) ) ;
#8299=CARTESIAN_POINT ( 'NONE',  ( 1.530808498934191521E-15, 3.862499998088169573, -25.00000000000000000 ) ) ;
#8302=CARTESIAN_POINT ( 'NONE',  ( 15.13990010960492505, -0.001000000000001000089, 5.276923788646651126 ) ) ;
#8304=ORIENTED_EDGE ( 'NONE', *, *, #1320, .T. ) ;
#8305=ORIENTED_EDGE ( 'NONE', *, *, #2943, .T. ) ;
#8306=CIRCLE ( 'NONE', #4807, 25.00000000000000000 ) ;
#8307=ORIENTED_EDGE ( 'NONE', *, *, #916, .F. ) ;
#8312=DIRECTION ( 'NONE',  ( 0.000000000000000000, 1.000000000000000000, 0.000000000000000000 ) ) ;
#8317=ORIENTED_EDGE ( 'NONE', *, *, #778, .T. ) ;
#8320=CYLINDRICAL_SURFACE ( 'NONE', #5834, 2.999999999999999112 ) ;
#8321=CARTESIAN_POINT ( 'NONE',  ( 10.47307621135324496, 25.00000000000000000, -12.13990010960497479 ) ) ;
#8323=AXIS2_PLACEMENT_3D ( 'NONE', #2350, #9191, #5730 ) ;
#8329=CARTESIAN_POINT ( 'NONE',  ( -17.40975659021753330, 0.8437499990440846531, 17.40975659021752975 ) ) ;
#8333=AXIS2_PLACEMENT_3D ( 'NONE', #8446, #9395, #10115 ) ;
#8338=DIRECTION ( 'NONE',  ( 0.8660254037844398178, 0.000000000000000000, 0.4999999999999977796 ) ) ;
#8339=CARTESIAN_POINT ( 'NONE',  ( 24.62111388750000174, 0.2187499990440845699, 0.000000000000000000 ) ) ;
#8342=CARTESIAN_POINT ( 'NONE',  ( 0.000000000000000000, 28.00000000000000000, 0.000000000000000000 ) ) ;
#8344=EDGE_CURVE ( 'NONE', #7557, #5770, #10738, .T. ) ;
#8349=CARTESIAN_POINT ( 'NONE',  ( -5.276923788646812774, 28.00000000000000000, -15.13990010960486821 ) ) ;
#8350=AXIS2_PLACEMENT_3D ( 'NONE', #9090, #3970, #9707 ) ;
#8352=EDGE_CURVE ( 'NONE', #7304, #5695, #1608, .T. ) ;
#8357=CARTESIAN_POINT ( 'NONE',  ( -25.00000000000001421, 5.174999998088170017, 10.35533905932737397 ) ) ;
#8358=CARTESIAN_POINT ( 'NONE',  ( -17.40975659021752975, 0.5937499990440846531, -17.40975659021752975 ) ) ;
#8366=EDGE_LOOP ( 'NONE', ( #4999, #6663, #5472, #3023 ) ) ;
#8367=ORIENTED_EDGE ( 'NONE', *, *, #7163, .T. ) ;
#8370=ORIENTED_EDGE ( 'NONE', *, *, #10640, .T. ) ;
#8372=LINE ( 'NONE', #8421, #3952 ) ;
#8379=VERTEX_POINT ( 'NONE', #3842 ) ;
#8380=DIRECTION ( 'NONE',  ( -1.000000000000000000, 0.000000000000000000, 2.168404344971010347E-16 ) ) ;
#8382=DIRECTION ( 'NONE',  ( -0.000000000000000000, 1.000000000000000000, 0.000000000000000000 ) ) ;
#8383=LINE ( 'NONE', #1590, #7122 ) ;
#8384=CARTESIAN_POINT ( 'NONE',  ( 24.62111388750000174, 3.281249999044084653, -10.19839929293505776 ) ) ;
#8386=ORIENTED_EDGE ( 'NONE', *, *, #8828, .F. ) ;
#8388=CARTESIAN_POINT ( 'NONE',  ( 1.507608415688466075E-15, 2.468749999044085097, -24.62111388750000174 ) ) ;
#8390=EDGE_LOOP ( 'NONE', ( #2662, #767, #4703, #1076, #989 ) ) ;
#8399=EDGE_LOOP ( 'NONE', ( #7648, #10107 ) ) ;
#8400=EDGE_CURVE ( 'NONE', #7041, #1422, #1265, .T. ) ;
#8401=DIRECTION ( 'NONE',  ( -0.000000000000000000, 1.000000000000000000, -0.000000000000000000 ) ) ;
#8403=CARTESIAN_POINT ( 'NONE',  ( 17.67766952966368521, 5.487499998088169129, 17.67766952966369232 ) ) ;
#8404=CARTESIAN_POINT ( 'NONE',  ( -4.522825247065398226E-15, 1.968749999044084653, 24.62111388750000174 ) ) ;
#8406=ORIENTED_EDGE ( 'NONE', *, *, #2455, .T. ) ;
#8421=CARTESIAN_POINT ( 'NONE',  ( -2.999999999999996447, -0.001000000000001000089, 19.75000000000000000 ) ) ;
#8425=VECTOR ( 'NONE', #9901, 1000.000000000000000 ) ;
#8426=EDGE_CURVE ( 'NONE', #8118, #4659, #8868, .T. ) ;
#8431=CARTESIAN_POINT ( 'NONE',  ( 0.000000000000000000, 28.00000000000000000, 0.000000000000000000 ) ) ;
#8435=CIRCLE ( 'NONE', #1555, 2.999999999999997335 ) ;
#8437=FACE_OUTER_BOUND ( 'NONE', #3657, .T. ) ;
#8441=CARTESIAN_POINT ( 'NONE',  ( -10.19839929293507552, 4.906249999044083765, 24.62111388749999463 ) ) ;
#8443=ORIENTED_EDGE ( 'NONE', *, *, #931, .F. ) ;
#8446=CARTESIAN_POINT ( 'NONE',  ( 0.000000000000000000, 85.00000000000000000, 0.000000000000000000 ) ) ;
#8450=VECTOR ( 'NONE', #6862, 1000.000000000000000 ) ;
#8455=ADVANCED_FACE ( 'NONE', ( #424 ), #10528, .F. ) ;
#8458=CARTESIAN_POINT ( 'NONE',  ( -10.19839929293507552, 3.906249999044085097, 24.62111388749999463 ) ) ;
#8460=AXIS2_PLACEMENT_3D ( 'NONE', #10934, #1701, #6738 ) ;
#8465=CARTESIAN_POINT ( 'NONE',  ( 0.000000000000000000, 85.00000000000000000, 0.000000000000000000 ) ) ;
#8467=ORIENTED_EDGE ( 'NONE', *, *, #4982, .T. ) ;
#8469=ORIENTED_EDGE ( 'NONE', *, *, #6280, .F. ) ;
#8475=CARTESIAN_POINT ( 'NONE',  ( -7.874999999999821476, 25.00000000000000000, 13.63990010960501031 ) ) ;
#8478=DIRECTION ( 'NONE',  ( 0.000000000000000000, 1.000000000000000000, 0.000000000000000000 ) ) ;
#8480=AXIS2_PLACEMENT_3D ( 'NONE', #170, #9515, #1009 ) ;
#8482=CARTESIAN_POINT ( 'NONE',  ( 2.999999999999996447, -0.001000000000001000089, -19.75000000000000000 ) ) ;
#8495=CARTESIAN_POINT ( 'NONE',  ( -4.522825247065398226E-15, 4.968749999044083765, 24.62111388750000174 ) ) ;
#8496=AXIS2_PLACEMENT_3D ( 'NONE', #6481, #9837, #7248 ) ;
#8497=AXIS2_PLACEMENT_3D ( 'NONE', #4959, #6554, #1690 ) ;
#8500=CARTESIAN_POINT ( 'NONE',  ( 17.67766952966368521, 2.875000000000000000, 17.67766952966369232 ) ) ;
#8501=FACE_OUTER_BOUND ( 'NONE', #5364, .T. ) ;
#8503=CYLINDRICAL_SURFACE ( 'NONE', #7094, 2.999999999999997335 ) ;
#8507=DIRECTION ( 'NONE',  ( 0.000000000000000000, 0.000000000000000000, 1.000000000000000000 ) ) ;
#8509=AXIS2_PLACEMENT_3D ( 'NONE', #4534, #3680, #2835 ) ;
#8514=VECTOR ( 'NONE', #9132, 1000.000000000000000 ) ;
#8515=DIRECTION ( 'NONE',  ( 0.000000000000000000, 0.000000000000000000, -1.000000000000000000 ) ) ;
#8517=CARTESIAN_POINT ( 'NONE',  ( 10.19839929293505953, 0.5812499990440845865, -24.62111388750000174 ) ) ;
#8519=CARTESIAN_POINT ( 'NONE',  ( -4.592425496802574367E-15, 5.362499998088169129, 25.00000000000000000 ) ) ;
#8521=CARTESIAN_POINT ( 'NONE',  ( 1.530808498934191521E-15, 1.250000000000000000, -25.00000000000000000 ) ) ;
#8522=SURFACE_STYLE_FILL_AREA ( #5172 ) ;
#8523=ORIENTED_EDGE ( 'NONE', *, *, #921, .T. ) ;
#8525=FACE_BOUND ( 'NONE', #10360, .T. ) ;
#8526=DIRECTION ( 'NONE',  ( -0.000000000000000000, -1.000000000000000000, -0.000000000000000000 ) ) ;
#8530=ORIENTED_EDGE ( 'NONE', *, *, #1407, .F. ) ;
#8531=ORIENTED_EDGE ( 'NONE', *, *, #5837, .F. ) ;
#8532=ORIENTED_EDGE ( 'NONE', *, *, #9761, .F. ) ;
#8536=CARTESIAN_POINT ( 'NONE',  ( 3.957930336368489021E-15, 28.00000000000000000, 22.75000000000000000 ) ) ;
#8537=DIRECTION ( 'NONE',  ( -0.000000000000000000, 1.000000000000000000, -0.000000000000000000 ) ) ;
#8538=EDGE_CURVE ( 'NONE', #8662, #2067, #5497, .T. ) ;
#8540=EDGE_CURVE ( 'NONE', #5295, #10359, #1986, .T. ) ;
#8541=LINE ( 'NONE', #4298, #2457 ) ;
#8545=ORIENTED_EDGE ( 'NONE', *, *, #9107, .T. ) ;
#8547=DIRECTION ( 'NONE',  ( 1.156482317317872514E-15, 0.000000000000000000, 1.000000000000000000 ) ) ;
#8550=DIRECTION ( 'NONE',  ( 0.000000000000000000, 1.000000000000000000, 0.000000000000000000 ) ) ;
#8552=CARTESIAN_POINT ( 'NONE',  ( -25.00000000000000000, 5.049999998088170017, -10.35533905932738108 ) ) ;
#8553=EDGE_CURVE ( 'NONE', #5726, #4087, #5822, .T. ) ;
#8554=CARTESIAN_POINT ( 'NONE',  ( 10.19839929293505953, 4.406249999044084653, -24.62111388750000174 ) ) ;
#8555=EDGE_CURVE ( 'NONE', #1673, #1427, #3739, .T. ) ;
#8558=CARTESIAN_POINT ( 'NONE',  ( 25.00000000000000000, 3.000000000000000000, 0.000000000000000000 ) ) ;
#8559=FACE_OUTER_BOUND ( 'NONE', #4341, .T. ) ;
#8561=CARTESIAN_POINT ( 'NONE',  ( -17.67766952966368876, 3.375000000000000000, -17.67766952966369232 ) ) ;
#8563=DIRECTION ( 'NONE',  ( 0.000000000000000000, 1.000000000000000000, 0.000000000000000000 ) ) ;
#8564=FACE_BOUND ( 'NONE', #9520, .T. ) ;
#8568=VERTEX_POINT ( 'NONE', #8299 ) ;
#8570=EDGE_LOOP ( 'NONE', ( #5674, #4038, #714, #10079 ) ) ;
#8571=DIRECTION ( 'NONE',  ( -0.000000000000000000, 1.000000000000000000, -0.000000000000000000 ) ) ;
#8574=CARTESIAN_POINT ( 'NONE',  ( 17.67766952966369232, 2.737499998088169573, -17.67766952966369232 ) ) ;
#8575=CARTESIAN_POINT ( 'NONE',  ( 25.00000000000000000, -2.710505431213761085E-17, 0.000000000000000000 ) ) ;
#8583=CARTESIAN_POINT ( 'NONE',  ( 18.60400172474268032, 28.00000000000000000, 7.276923788646641356 ) ) ;
#8584=ORIENTED_EDGE ( 'NONE', *, *, #439, .F. ) ;
#8597=CARTESIAN_POINT ( 'NONE',  ( 17.40975659021752620, 5.268749999044085364, 17.40975659021753330 ) ) ;
#8599=EDGE_LOOP ( 'NONE', ( #198, #2800, #7266, #8739 ) ) ;
#8607=DIRECTION ( 'NONE',  ( -0.000000000000000000, 1.000000000000000000, 0.000000000000000000 ) ) ;
#8609=CARTESIAN_POINT ( 'NONE',  ( -17.40975659021752975, 3.593749999044084653, -17.40975659021752975 ) ) ;
#8610=EDGE_CURVE ( 'NONE', #3100, #7830, #6223, .T. ) ;
#8611=VECTOR ( 'NONE', #10353, 1000.000000000000000 ) ;
#8619=CARTESIAN_POINT ( 'NONE',  ( -24.62111388750000884, 1.956249999044084698, 10.19839929293505421 ) ) ;
#8625=ADVANCED_FACE ( 'NONE', ( #6054 ), #8638, .F. ) ;
#8626=ORIENTED_EDGE ( 'NONE', *, *, #7163, .F. ) ;
#8627=ORIENTED_EDGE ( 'NONE', *, *, #4721, .T. ) ;
#8631=CARTESIAN_POINT ( 'NONE',  ( 10.35533905932737930, 3.799999998088170017, -25.00000000000000000 ) ) ;
#8632=CARTESIAN_POINT ( 'NONE',  ( -10.19839929293505776, 4.531249999044084653, -24.62111388750000174 ) ) ;
#8633=LINE ( 'NONE', #10180, #7366 ) ;
#8637=FACE_BOUND ( 'NONE', #4012, .T. ) ;
#8638=CYLINDRICAL_SURFACE ( 'NONE', #3169, 2.999999999999997335 ) ;
#8639=CARTESIAN_POINT ( 'NONE',  ( -7.276923788646840308, 25.00000000000000000, -18.60400172474260216 ) ) ;
#8643=ORIENTED_EDGE ( 'NONE', *, *, #520, .F. ) ;
#8644=ORIENTED_EDGE ( 'NONE', *, *, #2914, .T. ) ;
#8650=AXIS2_PLACEMENT_3D ( 'NONE', #3727, #5288, #10467 ) ;
#8652=CARTESIAN_POINT ( 'NONE',  ( 24.81055694375000087, 5.109374999522041882, 0.000000000000000000 ) ) ;
#8654=DIRECTION ( 'NONE',  ( 0.8660254037844399289, 0.000000000000000000, 0.4999999999999977796 ) ) ;
#8655=CARTESIAN_POINT ( 'NONE',  ( 2.143131898507867459E-15, 8.000000000000000000, -15.00000000000000178 ) ) ;
#8658=VECTOR ( 'NONE', #5647, 1000.000000000000000 ) ;
#8659=( BOUNDED_SURFACE ( )  B_SPLINE_SURFACE ( 1, 2, ( 
 ( #5491, #510, #2927, #8854, #7199, #1297, #410, #2975, #3784, #2216, #3880, #9012, #4679, #1438, #3996, #4832, #2166, #616, #8029, #6383, #5549, #8908, #10724, #1342, #9526, #6941, #6220, #10350, #2713, #9470, #7875, #6109, #1963, #2021, #8574, #298, #3663, #6162, #7815, #7046, #5336, #248, #6878, #8750, #10404, #1140, #2822, #8694, #4520, #1902, #5283, #8631, #5393, #186, #9581, #10299, #1188, #1080, #1848, #4569, #2651, #10236, #6049, #9408, #5231, #7754, #1023, #4456, #3606, #6994, #2763, #4392, #3546, #8357, #7475, #5002, #8519, #5814, #8403, #4164, #3429 ),
 ( #9124, #10128, #10009, #3305, #9, #10178, #10851, #10905, #5106, #8294, #3249, #7577, #6768, #127, #971, #9233, #9285, #4274, #2596, #2540, #10068, #5990, #4335, #906, #846, #5933, #7526, #4214, #6708, #5059, #7638, #2434, #74, #5758, #6821, #9345, #1789, #5170, #7698, #2483, #3488, #6648, #9178, #9954, #2385, #4943, #5879, #735, #798, #1677, #316, #6967, #1985, #1208, #269, #1924, #152, #10372, #6904, #8769, #10425, #5305, #4354, #1103, #7938, #9547, #10260, #6077, #2785, #4483, #9490, #6181, #6244, #2842, #3572, #5252, #10323, #2037, #8597, #7895, #5361 ) ),
 .UNSPECIFIED., .F., .F., .F. ) 
 B_SPLINE_SURFACE_WITH_KNOTS ( ( 2, 2 ),
 ( 3, 2, 2, 2, 2, 2, 2, 2, 2, 2, 2, 2, 2, 2, 2, 2, 2, 2, 2, 2, 2, 2, 2, 2, 2, 2, 2, 2, 2, 2, 2, 2, 2, 2, 2, 2, 2, 2, 2, 2, 3 ),
 ( 0.000000000000000000, 1.000000000000000000 ),
 ( 0.000000000000000000, 0.02500000000000000139, 0.05000000000000000278, 0.07499999999999999722, 0.1000000000000000056, 0.1250000000000000000, 0.1499999999999999944, 0.1749999999999999889, 0.2000000000000000111, 0.2250000000000000056, 0.2500000000000000000, 0.2750000000000000222, 0.2999999999999999889, 0.3250000000000000111, 0.3499999999999999778, 0.3750000000000000000, 0.4000000000000000222, 0.4249999999999999889, 0.4500000000000000111, 0.4749999999999999778, 0.5000000000000000000, 0.5250000000000000222, 0.5500000000000000444, 0.5749999999999999556, 0.5999999999999999778, 0.6250000000000000000, 0.6500000000000000222, 0.6750000000000000444, 0.6999999999999999556, 0.7249999999999999778, 0.7500000000000000000, 0.7750000000000000222, 0.8000000000000000444, 0.8249999999999999556, 0.8499999999999999778, 0.8750000000000000000, 0.9000000000000000222, 0.9250000000000000444, 0.9499999999999999556, 0.9749999999999999778, 1.000000000000000000 ),
 .UNSPECIFIED. ) 
 GEOMETRIC_REPRESENTATION_ITEM ( )  RATIONAL_B_SPLINE_SURFACE ( (
 ( 1.000000000000000000, 0.9238795325112867385, 1.000000000000000000, 0.9238795325112867385, 1.000000000000000000, 0.9238795325112867385, 1.000000000000000000, 0.9238795325112867385, 1.000000000000000000, 0.9238795325112867385, 1.000000000000000000, 0.9238795325112867385, 1.000000000000000000, 0.9238795325112867385, 1.000000000000000000, 0.9238795325112867385, 1.000000000000000000, 0.9238795325112867385, 1.000000000000000000, 0.9238795325112867385, 1.000000000000000000, 0.9238795325112867385, 1.000000000000000000, 0.9238795325112867385, 1.000000000000000000, 0.9238795325112867385, 1.000000000000000000, 0.9238795325112867385, 1.000000000000000000, 0.9238795325112867385, 1.000000000000000000, 0.9238795325112867385, 1.000000000000000000, 0.9238795325112867385, 1.000000000000000000, 0.9238795325112867385, 1.000000000000000000, 0.9238795325112867385, 1.000000000000000000, 0.9238795325112867385, 1.000000000000000000, 0.9238795325112867385, 1.000000000000000000, 0.9238795325112867385, 1.000000000000000000, 0.9238795325112867385, 1.000000000000000000, 0.9238795325112867385, 1.000000000000000000, 0.9238795325112867385, 1.000000000000000000, 0.9238795325112867385, 1.000000000000000000, 0.9238795325112867385, 1.000000000000000000, 0.9238795325112867385, 1.000000000000000000, 0.9238795325112867385, 1.000000000000000000, 0.9238795325112867385, 1.000000000000000000, 0.9238795325112867385, 1.000000000000000000, 0.9238795325112867385, 1.000000000000000000, 0.9238795325112867385, 1.000000000000000000, 0.9238795325112867385, 1.000000000000000000, 0.9238795325112867385, 1.000000000000000000, 0.9238795325112867385, 1.000000000000000000, 0.9238795325112867385, 1.000000000000000000, 0.9238795325112867385, 1.000000000000000000, 0.9238795325112867385, 1.000000000000000000, 0.9238795325112867385, 1.000000000000000000),
 ( 1.000000000000000000, 0.9238795325112867385, 1.000000000000000000, 0.9238795325112867385, 1.000000000000000000, 0.9238795325112867385, 1.000000000000000000, 0.9238795325112867385, 1.000000000000000000, 0.9238795325112867385, 1.000000000000000000, 0.9238795325112867385, 1.000000000000000000, 0.9238795325112867385, 1.000000000000000000, 0.9238795325112867385, 1.000000000000000000, 0.9238795325112867385, 1.000000000000000000, 0.9238795325112867385, 1.000000000000000000, 0.9238795325112867385, 1.000000000000000000, 0.9238795325112867385, 1.000000000000000000, 0.9238795325112867385, 1.000000000000000000, 0.9238795325112867385, 1.000000000000000000, 0.9238795325112867385, 1.000000000000000000, 0.9238795325112867385, 1.000000000000000000, 0.9238795325112867385, 1.000000000000000000, 0.9238795325112867385, 1.000000000000000000, 0.9238795325112867385, 1.000000000000000000, 0.9238795325112867385, 1.000000000000000000, 0.9238795325112867385, 1.000000000000000000, 0.9238795325112867385, 1.000000000000000000, 0.9238795325112867385, 1.000000000000000000, 0.9238795325112867385, 1.000000000000000000, 0.9238795325112867385, 1.000000000000000000, 0.9238795325112867385, 1.000000000000000000, 0.9238795325112867385, 1.000000000000000000, 0.9238795325112867385, 1.000000000000000000, 0.9238795325112867385, 1.000000000000000000, 0.9238795325112867385, 1.000000000000000000, 0.9238795325112867385, 1.000000000000000000, 0.9238795325112867385, 1.000000000000000000, 0.9238795325112867385, 1.000000000000000000, 0.9238795325112867385, 1.000000000000000000, 0.9238795325112867385, 1.000000000000000000, 0.9238795325112867385, 1.000000000000000000, 0.9238795325112867385, 1.000000000000000000, 0.9238795325112867385, 1.000000000000000000, 0.9238795325112867385, 1.000000000000000000, 0.9238795325112867385, 1.000000000000000000) ) ) 
 REPRESENTATION_ITEM ( '' )  SURFACE ( )  );
#8661=ORIENTED_EDGE ( 'NONE', *, *, #261, .T. ) ;
#8662=VERTEX_POINT ( 'NONE', #7879 ) ;
#8669=CARTESIAN_POINT ( 'NONE',  ( 3.957930336368489021E-15, 25.00000000000000000, 22.75000000000000000 ) ) ;
#8671=LINE ( 'NONE', #1114, #751 ) ;
#8678=VERTEX_POINT ( 'NONE', #5399 ) ;
#8683=AXIS2_PLACEMENT_3D ( 'NONE', #2378, #10118, #8283 ) ;
#8685=EDGE_CURVE ( 'NONE', #5242, #10312, #10185, .T. ) ;
#8687=ORIENTED_EDGE ( 'NONE', *, *, #9761, .T. ) ;
#8688=ORIENTED_EDGE ( 'NONE', *, *, #8947, .F. ) ;
#8692=AXIS2_PLACEMENT_3D ( 'NONE', #2077, #6903, #7066 ) ;
#8693=CARTESIAN_POINT ( 'NONE',  ( 25.00000000000000000, 0.6124999980881691286, 0.000000000000000000 ) ) ;
#8694=CARTESIAN_POINT ( 'NONE',  ( 24.99999999999999289, 3.549999998088169573, 10.35533905932739529 ) ) ;
#8695=CARTESIAN_POINT ( 'NONE',  ( -24.62111388750000174, 4.718749999044084653, -3.015216831376932151E-15 ) ) ;
#8696=VECTOR ( 'NONE', #5945, 999.9999999999998863 ) ;
#8700=DIRECTION ( 'NONE',  ( 8.881784197001254296E-16, 0.000000000000000000, 1.000000000000000000 ) ) ;
#8703=DIRECTION ( 'NONE',  ( -9.251858538542978533E-15, 0.000000000000000000, 1.000000000000000000 ) ) ;
#8710=CIRCLE ( 'NONE', #5880, 2.999999999999996891 ) ;
#8713=EDGE_CURVE ( 'NONE', #8678, #5068, #1087, .T. ) ;
#8714=LINE ( 'NONE', #10315, #10096 ) ;
#8716=CARTESIAN_POINT ( 'NONE',  ( 15.60400172474269453, -0.001000000000001000089, 12.47307621135327693 ) ) ;
#8719=DIRECTION ( 'NONE',  ( -0.000000000000000000, -1.000000000000000000, -0.000000000000000000 ) ) ;
#8720=DIRECTION ( 'NONE',  ( 0.000000000000000000, 1.000000000000000000, 0.000000000000000000 ) ) ;
#8722=ORIENTED_EDGE ( 'NONE', *, *, #6350, .T. ) ;
#8724=EDGE_LOOP ( 'NONE', ( #7386, #6562, #7613, #7587 ) ) ;
#8725=CARTESIAN_POINT ( 'NONE',  ( -4.592425496802574367E-15, 4.750000000000000000, 25.00000000000000000 ) ) ;
#8729=CYLINDRICAL_SURFACE ( 'NONE', #10300, 25.00000000000000000 ) ;
#8731=( BOUNDED_CURVE ( )  B_SPLINE_CURVE ( 2, ( #7917, #8944, #2868, #7968, #3769, #10504, #1376, #6265, #4761 ),
 .UNSPECIFIED., .F., .F. ) 
 B_SPLINE_CURVE_WITH_KNOTS ( ( 3, 2, 2, 2, 3 ),
 ( 0.3499999999999999778, 0.3750000000000000000, 0.4000000000000000222, 0.4249999999999999889, 0.4500000000000000111 ),
 .UNSPECIFIED. ) 
 CURVE ( )  GEOMETRIC_REPRESENTATION_ITEM ( )  RATIONAL_B_SPLINE_CURVE ( ( 1.000000000000000000, 0.9238795325112867385, 1.000000000000000000, 0.9238795325112867385, 1.000000000000000000, 0.9238795325112867385, 1.000000000000000000, 0.9238795325112867385, 1.000000000000000000 ) ) 
 REPRESENTATION_ITEM ( '' )  );
#8732=LINE ( 'NONE', #8004, #3037 ) ;
#8735=VERTEX_POINT ( 'NONE', #2600 ) ;
#8738=CARTESIAN_POINT ( 'NONE',  ( 24.62111388750000174, 1.393749999044084475, 0.000000000000000000 ) ) ;
#8739=ORIENTED_EDGE ( 'NONE', *, *, #2455, .F. ) ;
#8740=CARTESIAN_POINT ( 'NONE',  ( 18.60400172474263414, 25.00000000000000000, -7.276923788646775471 ) ) ;
#8741=CARTESIAN_POINT ( 'NONE',  ( 0.000000000000000000, 25.00000000000000000, -5.999999999999999112 ) ) ;
#8748=CARTESIAN_POINT ( 'NONE',  ( -4.522825247065398226E-15, 3.143749999044084475, 24.62111388750000174 ) ) ;
#8749=ADVANCED_FACE ( 'NONE', ( #5176 ), #975, .F. ) ;
#8750=CARTESIAN_POINT ( 'NONE',  ( -10.35533905932739174, 3.299999998088169129, 24.99999999999999289 ) ) ;
#8751=CARTESIAN_POINT ( 'NONE',  ( 25.00000000000000000, 2.000000000000000000, 0.000000000000000000 ) ) ;
#8753=CYLINDRICAL_SURFACE ( 'NONE', #7731, 2.999999999999997335 ) ;
#8755=CARTESIAN_POINT ( 'NONE',  ( 17.10400172474269098, -0.001000000000001000089, 9.874999999999957367 ) ) ;
#8759=EDGE_LOOP ( 'NONE', ( #3602, #4895, #10123, #8443 ) ) ;
#8760=ORIENTED_EDGE ( 'NONE', *, *, #778, .F. ) ;
#8761=CARTESIAN_POINT ( 'NONE',  ( 0.000000000000000000, 8.000000000000000000, 15.00000000000000178 ) ) ;
#8764=DIRECTION ( 'NONE',  ( -0.5000000000000012212, 0.000000000000000000, -0.8660254037844380415 ) ) ;
#8769=CARTESIAN_POINT ( 'NONE',  ( -10.19839929293507552, 4.081249999044084475, 24.62111388749999463 ) ) ;
#8774=FACE_OUTER_BOUND ( 'NONE', #9034, .T. ) ;
#8777=CARTESIAN_POINT ( 'NONE',  ( 13.63990010960487353, -0.001000000000001000089, -7.875000000000067502 ) ) ;
#8778=DIRECTION ( 'NONE',  ( 0.000000000000000000, 0.000000000000000000, 1.000000000000000000 ) ) ;
#8782=CIRCLE ( 'NONE', #2412, 2.999999999999996447 ) ;
#8784=CARTESIAN_POINT ( 'NONE',  ( 3.061616997868383043E-15, 85.00000000000000000, 25.00000000000000000 ) ) ;
#8788=DIRECTION ( 'NONE',  ( -0.8660254037844399289, 0.000000000000000000, -0.4999999999999977796 ) ) ;
#8789=VECTOR ( 'NONE', #1704, 1000.000000000000000 ) ;
#8791=LINE ( 'NONE', #345, #852 ) ;
#8792=ORIENTED_EDGE ( 'NONE', *, *, #469, .T. ) ;
#8797=CARTESIAN_POINT ( 'NONE',  ( -17.40975659021753330, 2.018749999044084475, 17.40975659021752975 ) ) ;
#8798=CARTESIAN_POINT ( 'NONE',  ( -17.67766952966369232, 2.625000000000000000, 17.67766952966368876 ) ) ;
#8804=CARTESIAN_POINT ( 'NONE',  ( -3.223142256880076948E-15, 25.00000000000000000, -15.75000000000000000 ) ) ;
#8806=EDGE_CURVE ( 'NONE', #448, #7899, #2111, .T. ) ;
#8808=FACE_BOUND ( 'NONE', #7649, .T. ) ;
#8810=CARTESIAN_POINT ( 'NONE',  ( -3.957930336368489021E-15, 28.00000000000000000, -19.75000000000000000 ) ) ;
#8812=CARTESIAN_POINT ( 'NONE',  ( 0.000000000000000000, 85.00000000000000000, 0.000000000000000000 ) ) ;
#8814=ORIENTED_EDGE ( 'NONE', *, *, #7971, .F. ) ;
#8822=CARTESIAN_POINT ( 'NONE',  ( -19.75000000000000000, 28.00000000000000000, 2.108281996628241301E-13 ) ) ;
#8828=EDGE_CURVE ( 'NONE', #2931, #5067, #8306, .T. ) ;
#8830=ORIENTED_EDGE ( 'NONE', *, *, #5831, .F. ) ;
#8832=EDGE_CURVE ( 'NONE', #857, #9220, #24, .T. ) ;
#8835=CARTESIAN_POINT ( 'NONE',  ( -4.592425496802574367E-15, 0.7500000000000000000, 25.00000000000000000 ) ) ;
#8837=ORIENTED_EDGE ( 'NONE', *, *, #636, .F. ) ;
#8838=PLANE ( 'NONE',  #189 ) ;
#8840=ORIENTED_EDGE ( 'NONE', *, *, #10924, .T. ) ;
#8844=EDGE_LOOP ( 'NONE', ( #10005, #464, #2492, #3165 ) ) ;
#8848=CARTESIAN_POINT ( 'NONE',  ( 1.507608415688466075E-15, 3.643749999044084920, -24.62111388750000174 ) ) ;
#8851=SURFACE_SIDE_STYLE ('',( #8522 ) ) ;
#8854=CARTESIAN_POINT ( 'NONE',  ( 10.35533905932737930, 0.7999999980881692396, -25.00000000000000000 ) ) ;
#8861=ORIENTED_EDGE ( 'NONE', *, *, #3060, .T. ) ;
#8867=AXIS2_PLACEMENT_3D ( 'NONE', #8716, #4537, #8654 ) ;
#8868=LINE ( 'NONE', #1308, #728 ) ;
#8871=LINE ( 'NONE', #8092, #6047 ) ;
#8872=VERTEX_POINT ( 'NONE', #3036 ) ;
#8877=EDGE_CURVE ( 'NONE', #9337, #3918, #217, .T. ) ;
#8879=CARTESIAN_POINT ( 'NONE',  ( 0.000000000000000000, 85.00000000000000000, 0.000000000000000000 ) ) ;
#8881=DIRECTION ( 'NONE',  ( 0.000000000000000000, 0.000000000000000000, 1.000000000000000000 ) ) ;
#8883=LINE ( 'NONE', #1317, #1999 ) ;
#8885=EDGE_CURVE ( 'NONE', #10673, #3501, #9786, .T. ) ;
#8888=EDGE_LOOP ( 'NONE', ( #4269, #8687, #4795, #10805 ) ) ;
#8892=ORIENTED_EDGE ( 'NONE', *, *, #4549, .F. ) ;
#8904=CARTESIAN_POINT ( 'NONE',  ( 10.19839929293506486, 3.206249999044084031, 24.62111388749999819 ) ) ;
#8905=CARTESIAN_POINT ( 'NONE',  ( 24.99999999999999289, 3.937500000000000000, 10.35533905932739529 ) ) ;
#8908=CARTESIAN_POINT ( 'NONE',  ( -10.35533905932737575, 1.924999998088169129, -25.00000000000000000 ) ) ;
#8916=CARTESIAN_POINT ( 'NONE',  ( 17.10400172474269098, -0.001000000000001000089, 9.874999999999957367 ) ) ;
#8917=DIRECTION ( 'NONE',  ( 0.8660254037844402619, -0.4999999999999970579, 0.000000000000000000 ) ) ;
#8918=DIRECTION ( 'NONE',  ( -0.000000000000000000, 1.000000000000000000, -0.000000000000000000 ) ) ;
#8919=CARTESIAN_POINT ( 'NONE',  ( 2.449293598294706513E-15, 20.00000000000000355, -20.00000000000000000 ) ) ;
#8922=ORIENTED_EDGE ( 'NONE', *, *, #1157, .T. ) ;
#8923=ORIENTED_EDGE ( 'NONE', *, *, #5600, .T. ) ;
#8931=ADVANCED_FACE ( 'NONE', ( #2976 ), #6384, .F. ) ;
#8932=ORIENTED_EDGE ( 'NONE', *, *, #8685, .T. ) ;
#8935=CARTESIAN_POINT ( 'NONE',  ( -9.874999999999777955, 28.00000000000000000, 17.10400172474279401 ) ) ;
#8936=CARTESIAN_POINT ( 'NONE',  ( -10.19839929293505776, 3.706249999044085808, -24.62111388750000174 ) ) ;
#8938=LINE ( 'NONE', #4756, #8987 ) ;
#8940=CARTESIAN_POINT ( 'NONE',  ( 0.000000000000000000, 25.00000000000000000, 0.000000000000000000 ) ) ;
#8944=CARTESIAN_POINT ( 'NONE',  ( 10.35533905932738286, 2.424999998088169129, 24.99999999999999645 ) ) ;
#8945=EDGE_LOOP ( 'NONE', ( #3133, #5580, #7364, #10393, #9809 ) ) ;
#8947=EDGE_CURVE ( 'NONE', #917, #8872, #6231, .T. ) ;
#8949=EDGE_CURVE ( 'NONE', #1513, #6058, #1436, .T. ) ;
#8950=CIRCLE ( 'NONE', #1209, 2.999999999999997335 ) ;
#8952=CARTESIAN_POINT ( 'NONE',  ( 15.74999999999999289, 25.00000000000000000, -3.000000000000053291 ) ) ;
#8953=CARTESIAN_POINT ( 'NONE',  ( 24.62111388749999463, 3.331249999044084920, 10.19839929293507730 ) ) ;
#8954=ORIENTED_EDGE ( 'NONE', *, *, #3392, .F. ) ;
#8955=CARTESIAN_POINT ( 'NONE',  ( -25.00000000000000000, 4.437500000000000888, -10.35533905932738108 ) ) ;
#8956=SURFACE_STYLE_USAGE ( .BOTH. , #8851 ) ;
#8958=DIRECTION ( 'NONE',  ( 0.000000000000000000, 1.000000000000000000, 0.000000000000000000 ) ) ;
#8959=CARTESIAN_POINT ( 'NONE',  ( -2.999999999999996447, 28.00000000000000000, 19.75000000000000000 ) ) ;
#8960=CARTESIAN_POINT ( 'NONE',  ( 25.00000000000000000, 1.062500000000000222, -10.35533905932737753 ) ) ;
#8964=ADVANCED_FACE ( 'NONE', ( #6641 ), #2533, .T. ) ;
#8974=LINE ( 'NONE', #1309, #4621 ) ;
#8977=ORIENTED_EDGE ( 'NONE', *, *, #1576, .T. ) ;
#8983=PLANE ( 'NONE',  #10121 ) ;
#8984=CARTESIAN_POINT ( 'NONE',  ( -13.63990010960498367, 25.00000000000000000, -4.874999999999871214 ) ) ;
#8986=AXIS2_PLACEMENT_3D ( 'NONE', #558, #1387, #4773 ) ;
#8987=VECTOR ( 'NONE', #8212, 1000.000000000000000 ) ;
#8988=LINE ( 'NONE', #7225, #9715 ) ;
#8991=CARTESIAN_POINT ( 'NONE',  ( -4.522825247065398226E-15, 3.143749999044084475, 24.62111388750000174 ) ) ;
#8998=CARTESIAN_POINT ( 'NONE',  ( 24.62111388749999108, 3.156249999044084653, 10.19839929293507730 ) ) ;
#8999=EDGE_LOOP ( 'NONE', ( #5928, #9943, #2590, #4487, #3887 ) ) ;
#9001=ORIENTED_EDGE ( 'NONE', *, *, #9661, .F. ) ;
#9006=CARTESIAN_POINT ( 'NONE',  ( -24.62111388750000174, 2.718749999044084653, -3.015216831376932151E-15 ) ) ;
#9007=CARTESIAN_POINT ( 'NONE',  ( 7.874999999999916511, 25.00000000000000000, -10.63990010960495702 ) ) ;
#9009=CIRCLE ( 'NONE', #8273, 2.999999999999999112 ) ;
#9012=CARTESIAN_POINT ( 'NONE',  ( -10.35533905932739174, 1.299999998088169129, 24.99999999999999289 ) ) ;
#9016=ORIENTED_EDGE ( 'NONE', *, *, #994, .T. ) ;
#9019=EDGE_CURVE ( 'NONE', #5067, #3964, #788, .T. ) ;
#9020=EDGE_LOOP ( 'NONE', ( #2300, #3166, #9724, #4918 ) ) ;
#9022=CARTESIAN_POINT ( 'NONE',  ( 0.000000000000000000, 8.000000000000003553, 0.000000000000000000 ) ) ;
#9031=EDGE_CURVE ( 'NONE', #7140, #10484, #7518, .T. ) ;
#9032=VECTOR ( 'NONE', #9948, 1000.000000000000000 ) ;
#9034=EDGE_LOOP ( 'NONE', ( #306, #9111, #9187, #181 ) ) ;
#9035=ADVANCED_FACE ( 'NONE', ( #3357, #6757 ), #5810, .T. ) ;
#9040=CYLINDRICAL_SURFACE ( 'NONE', #3380, 25.00000000000000000 ) ;
#9042=CARTESIAN_POINT ( 'NONE',  ( -2.999999999999996447, 28.00000000000000000, 19.75000000000000000 ) ) ;
#9048=CIRCLE ( 'NONE', #7274, 2.999999999999997780 ) ;
#9051=AXIS2_PLACEMENT_3D ( 'NONE', #5025, #1749, #4350 ) ;
#9053=CARTESIAN_POINT ( 'NONE',  ( 1.507608415688466075E-15, 4.643749999044084475, -24.62111388750000174 ) ) ;
#9054=ORIENTED_EDGE ( 'NONE', *, *, #8555, .F. ) ;
#9059=CARTESIAN_POINT ( 'NONE',  ( 24.62111388750000174, 0.2812499990440845421, -10.19839929293505776 ) ) ;
#9061=CONICAL_SURFACE ( 'NONE', #6590, 20.00000000000000000, 0.3947911196997613281 ) ;
#9062=ORIENTED_EDGE ( 'NONE', *, *, #119, .T. ) ;
#9066=CARTESIAN_POINT ( 'NONE',  ( -4.522825247065398226E-15, 5.143749999044084475, 24.62111388750000174 ) ) ;
#9068=CYLINDRICAL_SURFACE ( 'NONE', #1212, 2.999999999999997335 ) ;
#9069=DIRECTION ( 'NONE',  ( -0.000000000000000000, 1.000000000000000000, 0.000000000000000000 ) ) ;
#9071=CARTESIAN_POINT ( 'NONE',  ( 3.061616997868383043E-15, 85.00000000000000000, 25.00000000000000000 ) ) ;
#9075=EDGE_CURVE ( 'NONE', #2200, #652, #1501, .T. ) ;
#9078=LINE ( 'NONE', #5610, #5546 ) ;
#9080=CARTESIAN_POINT ( 'NONE',  ( -17.10400172474254532, 25.00000000000000000, 9.875000000000202505 ) ) ;
#9083=ORIENTED_EDGE ( 'NONE', *, *, #10855, .F. ) ;
#9086=ORIENTED_EDGE ( 'NONE', *, *, #10904, .T. ) ;
#9089=EDGE_CURVE ( 'NONE', #7005, #9938, #6040, .T. ) ;
#9090=CARTESIAN_POINT ( 'NONE',  ( 7.874999999999916511, 28.00000000000000000, -13.63990010960495702 ) ) ;
#9103=CARTESIAN_POINT ( 'NONE',  ( 1.507608415688466075E-15, 2.468749999044085097, -24.62111388750000174 ) ) ;
#9104=ORIENTED_EDGE ( 'NONE', *, *, #1525, .F. ) ;
#9107=EDGE_CURVE ( 'NONE', #2032, #963, #10492, .T. ) ;
#9110=CARTESIAN_POINT ( 'NONE',  ( -24.62111388750000884, 2.781249999044085541, 10.19839929293505421 ) ) ;
#9111=ORIENTED_EDGE ( 'NONE', *, *, #5799, .T. ) ;
#9116=DIRECTION ( 'NONE',  ( -0.5000000000000073275, 0.000000000000000000, -0.8660254037844344888 ) ) ;
#9117=LINE ( 'NONE', #10946, #7070 ) ;
#9121=ORIENTED_EDGE ( 'NONE', *, *, #5600, .F. ) ;
#9124=CARTESIAN_POINT ( 'NONE',  ( 24.62111388750000174, 0.3937499990440845310, 0.000000000000000000 ) ) ;
#9125=CARTESIAN_POINT ( 'NONE',  ( -10.19839929293507552, 1.906249999044084431, 24.62111388749999463 ) ) ;
#9126=DIRECTION ( 'NONE',  ( -0.000000000000000000, 1.000000000000000000, -0.000000000000000000 ) ) ;
#9129=DIRECTION ( 'NONE',  ( 0.000000000000000000, 1.000000000000000000, 0.000000000000000000 ) ) ;
#9132=DIRECTION ( 'NONE',  ( 0.000000000000000000, 1.000000000000000000, -0.000000000000000000 ) ) ;
#9134=ORIENTED_EDGE ( 'NONE', *, *, #9372, .F. ) ;
#9135=EDGE_LOOP ( 'NONE', ( #2916, #6830 ) ) ;
#9138=VECTOR ( 'NONE', #8571, 1000.000000000000000 ) ;
#9150=CARTESIAN_POINT ( 'NONE',  ( -7.874999999999821476, -0.001000000000001000089, 13.63990010960501031 ) ) ;
#9156=EDGE_CURVE ( 'NONE', #7557, #10846, #5504, .T. ) ;
#9157=CARTESIAN_POINT ( 'NONE',  ( -24.62111388750000174, 2.718749999044084653, -3.015216831376932151E-15 ) ) ;
#9158=ORIENTED_EDGE ( 'NONE', *, *, #10223, .T. ) ;
#9160=EDGE_CURVE ( 'NONE', #1567, #3209, #9613, .T. ) ;
#9164=DIRECTION ( 'NONE',  ( 0.4999999999999951705, 0.000000000000000000, -0.8660254037844413721 ) ) ;
#9165=CARTESIAN_POINT ( 'NONE',  ( -17.40975659021752975, 0.5937499990440846531, -17.40975659021752975 ) ) ;
#9169=FACE_OUTER_BOUND ( 'NONE', #10044, .T. ) ;
#9176=CIRCLE ( 'NONE', #7236, 2.999999999999996447 ) ;
#9178=CARTESIAN_POINT ( 'NONE',  ( -17.40975659021753330, 3.018749999044084475, 17.40975659021752975 ) ) ;
#9179=CARTESIAN_POINT ( 'NONE',  ( 24.62111388750000174, 0.2187499990440845699, 0.000000000000000000 ) ) ;
#9181=ORIENTED_EDGE ( 'NONE', *, *, #3491, .T. ) ;
#9187=ORIENTED_EDGE ( 'NONE', *, *, #7494, .T. ) ;
#9188=ORIENTED_EDGE ( 'NONE', *, *, #3817, .F. ) ;
#9191=DIRECTION ( 'NONE',  ( -0.5000000000000103251, 0.000000000000000000, -0.8660254037844327124 ) ) ;
#9194=DIRECTION ( 'NONE',  ( -0.000000000000000000, -1.000000000000000000, -0.000000000000000000 ) ) ;
#9200=CARTESIAN_POINT ( 'NONE',  ( 10.35533905932742016, 4.812499999999999112, 24.99999999999996447 ) ) ;
#9208=CARTESIAN_POINT ( 'NONE',  ( -4.522825247065398226E-15, 2.968749999044084653, 24.62111388750000174 ) ) ;
#9209=ADVANCED_FACE ( 'NONE', ( #7129 ), #5223, .F. ) ;
#9214=AXIS2_PLACEMENT_3D ( 'NONE', #8777, #1219, #4647 ) ;
#9218=CARTESIAN_POINT ( 'NONE',  ( -4.522825247065398226E-15, 1.968749999044084653, 24.62111388750000174 ) ) ;
#9220=VERTEX_POINT ( 'NONE', #961 ) ;
#9222=CARTESIAN_POINT ( 'NONE',  ( -4.592425496802574367E-15, 1.362499998088169129, 25.00000000000000000 ) ) ;
#9225=DIRECTION ( 'NONE',  ( 0.000000000000000000, 0.000000000000000000, -1.000000000000000000 ) ) ;
#9229=VERTEX_POINT ( 'NONE', #2088 ) ;
#9232=DIRECTION ( 'NONE',  ( -0.000000000000000000, -1.000000000000000000, -0.000000000000000000 ) ) ;
#9233=CARTESIAN_POINT ( 'NONE',  ( 24.62111388749999463, 1.331249999044084475, 10.19839929293507730 ) ) ;
#9234=CARTESIAN_POINT ( 'NONE',  ( -17.40975659021753330, 0.8437499990440846531, 17.40975659021752975 ) ) ;
#9243=ORIENTED_EDGE ( 'NONE', *, *, #2033, .T. ) ;
#9244=ORIENTED_EDGE ( 'NONE', *, *, #3926, .F. ) ;
#9259=LINE ( 'NONE', #6139, #8789 ) ;
#9263=ADVANCED_FACE ( 'NONE', ( #9711 ), #9330, .F. ) ;
#9267=DIRECTION ( 'NONE',  ( -3.708321773340234242E-15, 0.000000000000000000, -1.000000000000000000 ) ) ;
#9268=ORIENTED_EDGE ( 'NONE', *, *, #5846, .F. ) ;
#9269=LINE ( 'NONE', #3471, #8450 ) ;
#9272=CARTESIAN_POINT ( 'NONE',  ( -13.63990010960498367, 28.00000000000000000, -7.874999999999870326 ) ) ;
#9275=EDGE_CURVE ( 'NONE', #6044, #1816, #4326, .T. ) ;
#9277=EDGE_CURVE ( 'NONE', #5812, #120, #9807, .T. ) ;
#9278=ORIENTED_EDGE ( 'NONE', *, *, #3616, .T. ) ;
#9283=FACE_OUTER_BOUND ( 'NONE', #4544, .T. ) ;
#9284=( BOUNDED_SURFACE ( )  B_SPLINE_SURFACE ( 1, 2, ( 
 ( #9179, #6649, #6769, #1617, #4003, #624, #8358, #7476, #9955, #3250, #9234, #10069, #681, #2334, #4056, #5060, #5718, #7527, #799, #4165, #8191, #10852, #10906, #2484, #5881, #2386, #1678, #9125, #8404, #1558, #847, #4215, #4886, #7578, #7356, #3145, #6541, #8237, #10179, #249, #4336, #972, #6110, #3607, #2597, #10301, #6995, #6879, #6942, #7755, #9286, #2714, #5991, #3489, #187, #10351, #7640, #128, #1903, #8458, #3430, #3547, #9471, #299, #1142, #9410, #5284, #4457, #2764, #8632, #10237, #6163, #8695, #1081, #1024, #7816, #7699, #4393, #2652, #5232, #9527 ),
 ( #8575, #1964, #5337, #4521, #7876, #6050, #3664, #75, #9346, #10129, #2541, #5934, #1849, #1729, #5107, #907, #4275, #6822, #1790, #5171, #8521, #10516, #6221, #458, #2023, #5595, #7195, #7101, #3828, #10563, #8126, #2973, #8751, #5394, #6378, #9684, #3781, #8027, #3032, #3878, #5437, #10464, #8798, #9782, #2879, #1340, #9732, #2162, #6275, #4570, #4769, #5547, #9582, #6433, #4678, #407, #9632, #2060, #1189, #4720, #1237, #4620, #7923, #8905, #8073, #506, #7244, #10616, #7152, #2214, #7975, #8955, #2921, #6321, #1384, #3723, #555, #2107, #351, #7047, #10405 ) ),
 .UNSPECIFIED., .F., .F., .F. ) 
 B_SPLINE_SURFACE_WITH_KNOTS ( ( 2, 2 ),
 ( 3, 2, 2, 2, 2, 2, 2, 2, 2, 2, 2, 2, 2, 2, 2, 2, 2, 2, 2, 2, 2, 2, 2, 2, 2, 2, 2, 2, 2, 2, 2, 2, 2, 2, 2, 2, 2, 2, 2, 2, 3 ),
 ( 0.000000000000000000, 1.000000000000000000 ),
 ( 0.000000000000000000, 0.02500000000000000139, 0.05000000000000000278, 0.07499999999999999722, 0.1000000000000000056, 0.1250000000000000000, 0.1499999999999999944, 0.1749999999999999889, 0.2000000000000000111, 0.2250000000000000056, 0.2500000000000000000, 0.2750000000000000222, 0.2999999999999999889, 0.3250000000000000111, 0.3499999999999999778, 0.3750000000000000000, 0.4000000000000000222, 0.4249999999999999889, 0.4500000000000000111, 0.4749999999999999778, 0.5000000000000000000, 0.5250000000000000222, 0.5500000000000000444, 0.5749999999999999556, 0.5999999999999999778, 0.6250000000000000000, 0.6500000000000000222, 0.6750000000000000444, 0.6999999999999999556, 0.7249999999999999778, 0.7500000000000000000, 0.7750000000000000222, 0.8000000000000000444, 0.8249999999999999556, 0.8499999999999999778, 0.8750000000000000000, 0.9000000000000000222, 0.9250000000000000444, 0.9499999999999999556, 0.9749999999999999778, 1.000000000000000000 ),
 .UNSPECIFIED. ) 
 GEOMETRIC_REPRESENTATION_ITEM ( )  RATIONAL_B_SPLINE_SURFACE ( (
 ( 1.000000000000000000, 0.9238795325112867385, 1.000000000000000000, 0.9238795325112867385, 1.000000000000000000, 0.9238795325112867385, 1.000000000000000000, 0.9238795325112867385, 1.000000000000000000, 0.9238795325112867385, 1.000000000000000000, 0.9238795325112867385, 1.000000000000000000, 0.9238795325112867385, 1.000000000000000000, 0.9238795325112867385, 1.000000000000000000, 0.9238795325112867385, 1.000000000000000000, 0.9238795325112867385, 1.000000000000000000, 0.9238795325112867385, 1.000000000000000000, 0.9238795325112867385, 1.000000000000000000, 0.9238795325112867385, 1.000000000000000000, 0.9238795325112867385, 1.000000000000000000, 0.9238795325112867385, 1.000000000000000000, 0.9238795325112867385, 1.000000000000000000, 0.9238795325112867385, 1.000000000000000000, 0.9238795325112867385, 1.000000000000000000, 0.9238795325112867385, 1.000000000000000000, 0.9238795325112867385, 1.000000000000000000, 0.9238795325112867385, 1.000000000000000000, 0.9238795325112867385, 1.000000000000000000, 0.9238795325112867385, 1.000000000000000000, 0.9238795325112867385, 1.000000000000000000, 0.9238795325112867385, 1.000000000000000000, 0.9238795325112867385, 1.000000000000000000, 0.9238795325112867385, 1.000000000000000000, 0.9238795325112867385, 1.000000000000000000, 0.9238795325112867385, 1.000000000000000000, 0.9238795325112867385, 1.000000000000000000, 0.9238795325112867385, 1.000000000000000000, 0.9238795325112867385, 1.000000000000000000, 0.9238795325112867385, 1.000000000000000000, 0.9238795325112867385, 1.000000000000000000, 0.9238795325112867385, 1.000000000000000000, 0.9238795325112867385, 1.000000000000000000, 0.9238795325112867385, 1.000000000000000000, 0.9238795325112867385, 1.000000000000000000, 0.9238795325112867385, 1.000000000000000000, 0.9238795325112867385, 1.000000000000000000),
 ( 1.000000000000000000, 0.9238795325112867385, 1.000000000000000000, 0.9238795325112867385, 1.000000000000000000, 0.9238795325112867385, 1.000000000000000000, 0.9238795325112867385, 1.000000000000000000, 0.9238795325112867385, 1.000000000000000000, 0.9238795325112867385, 1.000000000000000000, 0.9238795325112867385, 1.000000000000000000, 0.9238795325112867385, 1.000000000000000000, 0.9238795325112867385, 1.000000000000000000, 0.9238795325112867385, 1.000000000000000000, 0.9238795325112867385, 1.000000000000000000, 0.9238795325112867385, 1.000000000000000000, 0.9238795325112867385, 1.000000000000000000, 0.9238795325112867385, 1.000000000000000000, 0.9238795325112867385, 1.000000000000000000, 0.9238795325112867385, 1.000000000000000000, 0.9238795325112867385, 1.000000000000000000, 0.9238795325112867385, 1.000000000000000000, 0.9238795325112867385, 1.000000000000000000, 0.9238795325112867385, 1.000000000000000000, 0.9238795325112867385, 1.000000000000000000, 0.9238795325112867385, 1.000000000000000000, 0.9238795325112867385, 1.000000000000000000, 0.9238795325112867385, 1.000000000000000000, 0.9238795325112867385, 1.000000000000000000, 0.9238795325112867385, 1.000000000000000000, 0.9238795325112867385, 1.000000000000000000, 0.9238795325112867385, 1.000000000000000000, 0.9238795325112867385, 1.000000000000000000, 0.9238795325112867385, 1.000000000000000000, 0.9238795325112867385, 1.000000000000000000, 0.9238795325112867385, 1.000000000000000000, 0.9238795325112867385, 1.000000000000000000, 0.9238795325112867385, 1.000000000000000000, 0.9238795325112867385, 1.000000000000000000, 0.9238795325112867385, 1.000000000000000000, 0.9238795325112867385, 1.000000000000000000, 0.9238795325112867385, 1.000000000000000000, 0.9238795325112867385, 1.000000000000000000, 0.9238795325112867385, 1.000000000000000000) ) ) 
 REPRESENTATION_ITEM ( '' )  SURFACE ( )  );
#9285=CARTESIAN_POINT ( 'NONE',  ( 24.62111388750000174, 1.393749999044084475, 0.000000000000000000 ) ) ;
#9286=CARTESIAN_POINT ( 'NONE',  ( 17.40975659021752975, 3.343749999044085097, -17.40975659021752975 ) ) ;
#9292=DIRECTION ( 'NONE',  ( -0.000000000000000000, 1.000000000000000000, 0.000000000000000000 ) ) ;
#9294=CIRCLE ( 'NONE', #1205, 2.999999999999999112 ) ;
#9295=ORIENTED_EDGE ( 'NONE', *, *, #855, .T. ) ;
#9296=ORIENTED_EDGE ( 'NONE', *, *, #3148, .T. ) ;
#9297=ORIENTED_EDGE ( 'NONE', *, *, #9624, .T. ) ;
#9299=ADVANCED_FACE ( 'NONE', ( #6560 ), #5680, .F. ) ;
#9301=DIRECTION ( 'NONE',  ( 0.000000000000000000, 0.000000000000000000, 1.000000000000000000 ) ) ;
#9304=DIRECTION ( 'NONE',  ( -0.000000000000000000, 1.000000000000000000, -0.000000000000000000 ) ) ;
#9306=CARTESIAN_POINT ( 'NONE',  ( 7.875000000000019540, 28.00000000000000000, 13.63990010960489840 ) ) ;
#9311=VERTEX_POINT ( 'NONE', #9760 ) ;
#9312=DIRECTION ( 'NONE',  ( 0.000000000000000000, 0.000000000000000000, 1.000000000000000000 ) ) ;
#9314=CARTESIAN_POINT ( 'NONE',  ( 3.957930336368489021E-15, -0.001000000000001000089, 19.75000000000000000 ) ) ;
#9319=CARTESIAN_POINT ( 'NONE',  ( -17.40975659021753330, 4.843749999044083765, 17.40975659021752975 ) ) ;
#9323=CARTESIAN_POINT ( 'NONE',  ( -4.592425496802574367E-15, 2.750000000000000000, 25.00000000000000000 ) ) ;
#9324=CARTESIAN_POINT ( 'NONE',  ( -19.75000000000003197, 28.00000000000000000, -2.999999999999789946 ) ) ;
#9330=CYLINDRICAL_SURFACE ( 'NONE', #9733, 2.999999999999997335 ) ;
#9331=LINE ( 'NONE', #5755, #3705 ) ;
#9332=PRODUCT_DEFINITION_SHAPE ( 'NONE', 'NONE',  #3451 ) ;
#9334=EDGE_LOOP ( 'NONE', ( #3193, #4253, #10862, #5180 ) ) ;
#9335=VECTOR ( 'NONE', #10000, 1000.000000000000000 ) ;
#9336=ORIENTED_EDGE ( 'NONE', *, *, #9156, .T. ) ;
#9337=VERTEX_POINT ( 'NONE', #4861 ) ;
#9340=FACE_OUTER_BOUND ( 'NONE', #3827, .T. ) ;
#9343=EDGE_CURVE ( 'NONE', #4087, #3378, #3219, .T. ) ;
#9344=ADVANCED_FACE ( 'NONE', ( #3063 ), #7221, .F. ) ;
#9345=CARTESIAN_POINT ( 'NONE',  ( 10.19839929293505953, 2.581249999044084475, -24.62111388750000174 ) ) ;
#9346=CARTESIAN_POINT ( 'NONE',  ( -25.00000000000000000, 0.5000000000000000000, -3.061616997868383043E-15 ) ) ;
#9347=DIRECTION ( 'NONE',  ( -0.000000000000000000, 1.000000000000000000, -0.000000000000000000 ) ) ;
#9352=FACE_BOUND ( 'NONE', #2444, .T. ) ;
#9353=DIRECTION ( 'NONE',  ( -0.000000000000000000, 1.000000000000000000, 0.000000000000000000 ) ) ;
#9355=CARTESIAN_POINT ( 'NONE',  ( 13.63990010960487353, -0.001000000000001000089, -4.875000000000070166 ) ) ;
#9359=ORIENTED_EDGE ( 'NONE', *, *, #7073, .T. ) ;
#9366=LINE ( 'NONE', #6724, #2175 ) ;
#9370=DIRECTION ( 'NONE',  ( -0.000000000000000000, 1.000000000000000000, -0.000000000000000000 ) ) ;
#9372=EDGE_CURVE ( 'NONE', #10596, #448, #7434, .T. ) ;
#9380=CARTESIAN_POINT ( 'NONE',  ( 15.60400172474260749, 28.00000000000000000, -12.47307621135338884 ) ) ;
#9381=DIRECTION ( 'NONE',  ( -0.000000000000000000, -1.000000000000000000, -0.000000000000000000 ) ) ;
#9383=DIRECTION ( 'NONE',  ( -0.000000000000000000, -1.000000000000000000, -0.000000000000000000 ) ) ;
#9384=DIRECTION ( 'NONE',  ( 0.000000000000000000, 0.000000000000000000, -1.000000000000000000 ) ) ;
#9387=AXIS2_PLACEMENT_3D ( 'NONE', #5244, #6175, #4411 ) ;
#9391=DIRECTION ( 'NONE',  ( -0.000000000000000000, -1.000000000000000000, -0.000000000000000000 ) ) ;
#9393=CARTESIAN_POINT ( 'NONE',  ( -25.00000000000001066, 3.562500000000000000, 10.35533905932737397 ) ) ;
#9394=AXIS2_PLACEMENT_3D ( 'NONE', #208, #7360, #7259 ) ;
#9395=DIRECTION ( 'NONE',  ( -0.000000000000000000, -1.000000000000000000, -0.000000000000000000 ) ) ;
#9396=AXIS2_PLACEMENT_3D ( 'NONE', #10594, #8101, #695 ) ;
#9397=CARTESIAN_POINT ( 'NONE',  ( -19.75000000000003197, -0.001000000000001000089, -2.999999999999789946 ) ) ;
#9402=ORIENTED_EDGE ( 'NONE', *, *, #5413, .F. ) ;
#9404=PLANE ( 'NONE',  #7055 ) ;
#9408=CARTESIAN_POINT ( 'NONE',  ( 24.99999999999999289, 4.549999998088169129, 10.35533905932739529 ) ) ;
#9409=CIRCLE ( 'NONE', #7462, 2.999999999999998668 ) ;
#9410=CARTESIAN_POINT ( 'NONE',  ( 24.62111388750000174, 4.281249999044084653, -10.19839929293505776 ) ) ;
#9414=FACE_BOUND ( 'NONE', #8945, .T. ) ;
#9417=CIRCLE ( 'NONE', #2171, 7.500000000000000888 ) ;
#9424=ORIENTED_EDGE ( 'NONE', *, *, #10595, .F. ) ;
#9425=ORIENTED_EDGE ( 'NONE', *, *, #7200, .F. ) ;
#9432=PLANE ( 'NONE',  #5522 ) ;
#9433=CYLINDRICAL_SURFACE ( 'NONE', #2127, 2.999999999999997335 ) ;
#9434=LINE ( 'NONE', #7779, #4652 ) ;
#9436=ORIENTED_EDGE ( 'NONE', *, *, #5455, .F. ) ;
#9439=EDGE_CURVE ( 'NONE', #9938, #3835, #8883, .T. ) ;
#9449=CARTESIAN_POINT ( 'NONE',  ( -24.62111388750000174, 3.718749999044084653, -3.015216831376932151E-15 ) ) ;
#9454=CARTESIAN_POINT ( 'NONE',  ( -4.522825247065398226E-15, 3.968749999044084209, 24.62111388750000174 ) ) ;
#9455=CARTESIAN_POINT ( 'NONE',  ( -24.62111388750000174, 1.831249999044084475, -10.19839929293506131 ) ) ;
#9456=ORIENTED_EDGE ( 'NONE', *, *, #10639, .T. ) ;
#9459=DIRECTION ( 'NONE',  ( -0.000000000000000000, 1.000000000000000000, 0.000000000000000000 ) ) ;
#9463=ORIENTED_EDGE ( 'NONE', *, *, #10430, .F. ) ;
#9467=DIRECTION ( 'NONE',  ( 0.000000000000000000, 0.000000000000000000, 1.000000000000000000 ) ) ;
#9470=CARTESIAN_POINT ( 'NONE',  ( 10.35533905932738286, 2.424999998088169129, 24.99999999999999645 ) ) ;
#9471=CARTESIAN_POINT ( 'NONE',  ( 17.40975659021752620, 4.093749999044084653, 17.40975659021753330 ) ) ;
#9477=CARTESIAN_POINT ( 'NONE',  ( 0.000000000000000000, 85.00000000000000000, 0.000000000000000000 ) ) ;
#9479=EDGE_LOOP ( 'NONE', ( #333, #6295 ) ) ;
#9481=VERTEX_POINT ( 'NONE', #4135 ) ;
#9485=CARTESIAN_POINT ( 'NONE',  ( 15.75000000000000000, -0.001000000000001000089, -5.821397334365942453E-14 ) ) ;
#9488=DIRECTION ( 'NONE',  ( 0.000000000000000000, 1.000000000000000000, 0.000000000000000000 ) ) ;
#9490=CARTESIAN_POINT ( 'NONE',  ( -17.40975659021752975, 4.768749999044084475, -17.40975659021752975 ) ) ;
#9499=ORIENTED_EDGE ( 'NONE', *, *, #6885, .T. ) ;
#9500=EDGE_CURVE ( 'NONE', #2327, #2786, #5951, .T. ) ;
#9505=CARTESIAN_POINT ( 'NONE',  ( -10.19839929293505776, 3.531249999044084653, -24.62111388750000174 ) ) ;
#9509=CARTESIAN_POINT ( 'NONE',  ( 15.75000000000001421, -0.001000000000001000089, 2.999999999999942268 ) ) ;
#9510=AXIS2_PLACEMENT_3D ( 'NONE', #5683, #4864, #3453 ) ;
#9511=CARTESIAN_POINT ( 'NONE',  ( -24.62111388750000174, 4.718749999044084653, -3.015216831376932151E-15 ) ) ;
#9514=EDGE_CURVE ( 'NONE', #5242, #8063, #10626, .T. ) ;
#9515=DIRECTION ( 'NONE',  ( 0.000000000000000000, 1.000000000000000000, 0.000000000000000000 ) ) ;
#9516=CARTESIAN_POINT ( 'NONE',  ( -25.00000000000000000, 2.437500000000000444, -10.35533905932738108 ) ) ;
#9517=FACE_BOUND ( 'NONE', #5757, .T. ) ;
#9520=EDGE_LOOP ( 'NONE', ( #4210, #3040, #7095, #4755, #6400 ) ) ;
#9526=CARTESIAN_POINT ( 'NONE',  ( -25.00000000000000000, 2.112499998088169129, -3.061616997868383043E-15 ) ) ;
#9527=CARTESIAN_POINT ( 'NONE',  ( 24.62111388750000174, 5.218749999044084653, 0.000000000000000000 ) ) ;
#9530=CARTESIAN_POINT ( 'NONE',  ( 20.00000000000000000, 20.00000000000000355, 0.000000000000000000 ) ) ;
#9536=ORIENTED_EDGE ( 'NONE', *, *, #9107, .F. ) ;
#9539=AXIS2_PLACEMENT_3D ( 'NONE', #10888, #780, #9990 ) ;
#9540=FACE_OUTER_BOUND ( 'NONE', #6333, .T. ) ;
#9541=VERTEX_POINT ( 'NONE', #5900 ) ;
#9543=PLANE ( 'NONE',  #8867 ) ;
#9547=CARTESIAN_POINT ( 'NONE',  ( 24.62111388750000174, 4.456249999044084475, -10.19839929293505776 ) ) ;
#9553=DIRECTION ( 'NONE',  ( -0.000000000000000000, -1.000000000000000000, -0.000000000000000000 ) ) ;
#9559=ORIENTED_EDGE ( 'NONE', *, *, #1452, .T. ) ;
#9560=EDGE_CURVE ( 'NONE', #4627, #7939, #746, .T. ) ;
#9562=CARTESIAN_POINT ( 'NONE',  ( 25.00000000000000000, 2.062500000000000000, -10.35533905932737753 ) ) ;
#9563=CARTESIAN_POINT ( 'NONE',  ( -25.00000000000000000, 0.5000000000000000000, -3.061616997868383043E-15 ) ) ;
#9569=CARTESIAN_POINT ( 'NONE',  ( 3.957930336368489021E-15, -0.001000000000001000089, 19.75000000000000000 ) ) ;
#9573=ADVANCED_FACE ( 'NONE', ( #9651 ), #315, .F. ) ;
#9575=ORIENTED_EDGE ( 'NONE', *, *, #8713, .T. ) ;
#9579=VECTOR ( 'NONE', #8160, 1000.000000000000000 ) ;
#9580=CARTESIAN_POINT ( 'NONE',  ( 10.19839929293505953, 3.581249999044085364, -24.62111388750000174 ) ) ;
#9581=CARTESIAN_POINT ( 'NONE',  ( -17.67766952966368876, 3.987499998088168685, -17.67766952966369232 ) ) ;
#9582=CARTESIAN_POINT ( 'NONE',  ( 1.530808498934191521E-15, 3.250000000000000444, -25.00000000000000000 ) ) ;
#9583=EDGE_CURVE ( 'NONE', #5968, #3303, #9434, .T. ) ;
#9585=CIRCLE ( 'NONE', #1118, 2.999999999999997335 ) ;
#9586=DIRECTION ( 'NONE',  ( 0.000000000000000000, -0.000000000000000000, -1.000000000000000000 ) ) ;
#9588=VECTOR ( 'NONE', #7176, 1000.000000000000000 ) ;
#9590=DIRECTION ( 'NONE',  ( -0.000000000000000000, -1.000000000000000000, -0.000000000000000000 ) ) ;
#9592=VERTEX_POINT ( 'NONE', #4417 ) ;
#9596=AXIS2_PLACEMENT_3D ( 'NONE', #7080, #483, #2798 ) ;
#9599=CARTESIAN_POINT ( 'NONE',  ( -19.74999999999996803, 25.00000000000000000, 3.000000000000206057 ) ) ;
#9601=CYLINDRICAL_SURFACE ( 'NONE', #2679, 2.999999999999999112 ) ;
#9610=CARTESIAN_POINT ( 'NONE',  ( 12.47307621135322186, -0.001000000000001000089, -15.60400172474273717 ) ) ;
#9613=LINE ( 'NONE', #5462, #7109 ) ;
#9614=ORIENTED_EDGE ( 'NONE', *, *, #8200, .T. ) ;
#9624=EDGE_CURVE ( 'NONE', #5481, #2342, #10804, .T. ) ;
#9626=ORIENTED_EDGE ( 'NONE', *, *, #8949, .T. ) ;
#9628=EDGE_CURVE ( 'NONE', #7410, #9311, #6759, .T. ) ;
#9631=CARTESIAN_POINT ( 'NONE',  ( -10.19839929293507552, 5.081249999044084475, 24.62111388749999463 ) ) ;
#9632=CARTESIAN_POINT ( 'NONE',  ( -25.00000000000000000, 3.500000000000000000, -3.061616997868383043E-15 ) ) ;
#9639=LINE ( 'NONE', #6226, #539 ) ;
#9646=CYLINDRICAL_SURFACE ( 'NONE', #2505, 2.999999999999999112 ) ;
#9651=FACE_OUTER_BOUND ( 'NONE', #5253, .T. ) ;
#9653=ADVANCED_FACE ( 'NONE', ( #1044 ), #3571, .F. ) ;
#9659=CARTESIAN_POINT ( 'NONE',  ( -10.47307621135315792, 25.00000000000000000, 12.13990010960504762 ) ) ;
#9661=EDGE_CURVE ( 'NONE', #6472, #4266, #1255, .T. ) ;
#9662=CIRCLE ( 'NONE', #6664, 2.999999999999996891 ) ;
#9663=VERTEX_POINT ( 'NONE', #7992 ) ;
#9664=VERTEX_POINT ( 'NONE', #6180 ) ;
#9668=CARTESIAN_POINT ( 'NONE',  ( -24.62111388750000174, 0.8312499990440843645, -10.19839929293506131 ) ) ;
#9669=ORIENTED_EDGE ( 'NONE', *, *, #4549, .T. ) ;
#9676=DIRECTION ( 'NONE',  ( -0.000000000000000000, 1.000000000000000000, -0.000000000000000000 ) ) ;
#9678=ORIENTED_EDGE ( 'NONE', *, *, #931, .T. ) ;
#9683=CARTESIAN_POINT ( 'NONE',  ( -24.62111388750000884, 3.956249999044084920, 10.19839929293505421 ) ) ;
#9684=CARTESIAN_POINT ( 'NONE',  ( 10.35533905932737930, 2.187500000000000444, -25.00000000000000000 ) ) ;
#9688=ORIENTED_EDGE ( 'NONE', *, *, #10452, .F. ) ;
#9690=LINE ( 'NONE', #5406, #6665 ) ;
#9697=CYLINDRICAL_SURFACE ( 'NONE', #6068, 2.999999999999999112 ) ;
#9703=VERTEX_POINT ( 'NONE', #2231 ) ;
#9706=EDGE_CURVE ( 'NONE', #4100, #634, #4286, .T. ) ;
#9707=DIRECTION ( 'NONE',  ( 0.4999999999999951705, 0.000000000000000000, -0.8660254037844413721 ) ) ;
#9709=CIRCLE ( 'NONE', #6720, 2.999999999999996891 ) ;
#9710=CARTESIAN_POINT ( 'NONE',  ( -15.60400172474278158, 25.00000000000000000, -12.47307621135316680 ) ) ;
#9711=FACE_OUTER_BOUND ( 'NONE', #3273, .T. ) ;
#9715=VECTOR ( 'NONE', #5630, 1000.000000000000000 ) ;
#9719=CARTESIAN_POINT ( 'NONE',  ( -24.62111388750000174, 3.831249999044084920, -10.19839929293506131 ) ) ;
#9722=CARTESIAN_POINT ( 'NONE',  ( 9.184850993605149917E-16, 31.00000000000000000, 7.500000000000000888 ) ) ;
#9724=ORIENTED_EDGE ( 'NONE', *, *, #7416, .F. ) ;
#9727=EDGE_LOOP ( 'NONE', ( #1195, #1912, #5161, #214 ) ) ;
#9731=CARTESIAN_POINT ( 'NONE',  ( -24.62111388750000174, 1.893749999044084475, -3.015216831376932151E-15 ) ) ;
#9732=CARTESIAN_POINT ( 'NONE',  ( 17.67766952966368521, 2.875000000000000000, 17.67766952966369232 ) ) ;
#9733=AXIS2_PLACEMENT_3D ( 'NONE', #3420, #6931, #8507 ) ;
#9735=CARTESIAN_POINT ( 'NONE',  ( -9.874999999999777955, -0.001000000000001000089, 17.10400172474279401 ) ) ;
#9736=CARTESIAN_POINT ( 'NONE',  ( 10.35533905932737930, 1.187500000000000000, -25.00000000000000000 ) ) ;
#9742=DIRECTION ( 'NONE',  ( -1.000000000000000000, 0.000000000000000000, 1.047444401652939533E-14 ) ) ;
#9748=EDGE_CURVE ( 'NONE', #7240, #3964, #5181, .T. ) ;
#9758=LINE ( 'NONE', #10491, #9588 ) ;
#9760=CARTESIAN_POINT ( 'NONE',  ( -4.592425496802574367E-15, 1.750000000000000000, 25.00000000000000000 ) ) ;
#9761=EDGE_CURVE ( 'NONE', #883, #10398, #8871, .T. ) ;
#9768=DIRECTION ( 'NONE',  ( 0.000000000000000000, 1.000000000000000000, -0.000000000000000000 ) ) ;
#9778=EDGE_CURVE ( 'NONE', #1422, #9950, #6395, .T. ) ;
#9781=CARTESIAN_POINT ( 'NONE',  ( -10.19839929293505776, 2.706249999044084475, -24.62111388750000174 ) ) ;
#9782=CARTESIAN_POINT ( 'NONE',  ( -10.35533905932739174, 2.687500000000000888, 24.99999999999999289 ) ) ;
#9786=LINE ( 'NONE', #7978, #4092 ) ;
#9794=CARTESIAN_POINT ( 'NONE',  ( -13.63990010960481492, -0.001000000000001000089, 7.875000000000163425 ) ) ;
#9795=FILL_AREA_STYLE_COLOUR ( '', #5609 ) ;
#9797=CARTESIAN_POINT ( 'NONE',  ( 3.061616997868383043E-15, 25.00000000000000000, 25.00000000000000000 ) ) ;
#9799=CARTESIAN_POINT ( 'NONE',  ( 0.000000000000000000, 25.00000000000000000, 0.000000000000000000 ) ) ;
#9801=ORIENTED_EDGE ( 'NONE', *, *, #1075, .F. ) ;
#9805=CARTESIAN_POINT ( 'NONE',  ( 0.000000000000000000, 31.00000000000000000, 0.000000000000000000 ) ) ;
#9807=LINE ( 'NONE', #1416, #935 ) ;
#9808=ORIENTED_EDGE ( 'NONE', *, *, #7843, .T. ) ;
#9809=ORIENTED_EDGE ( 'NONE', *, *, #5993, .F. ) ;
#9811=ADVANCED_FACE ( 'NONE', ( #2941 ), #9697, .F. ) ;
#9818=DIRECTION ( 'NONE',  ( 0.000000000000000000, 0.000000000000000000, 1.000000000000000000 ) ) ;
#9820=CARTESIAN_POINT ( 'NONE',  ( 7.874999999999916511, -0.001000000000001000089, -10.63990010960495880 ) ) ;
#9821=CARTESIAN_POINT ( 'NONE',  ( -24.62111388750000884, 0.7812499990440845421, 10.19839929293505421 ) ) ;
#9823=ORIENTED_EDGE ( 'NONE', *, *, #9706, .F. ) ;
#9829=FACE_OUTER_BOUND ( 'NONE', #3110, .T. ) ;
#9831=CARTESIAN_POINT ( 'NONE',  ( -4.522825247065398226E-15, 0.9687499990440845421, 24.62111388750000174 ) ) ;
#9837=DIRECTION ( 'NONE',  ( -0.000000000000000000, -1.000000000000000000, -0.000000000000000000 ) ) ;
#9838=CARTESIAN_POINT ( 'NONE',  ( 25.00000000000000000, 3.674999998088170017, -10.35533905932737753 ) ) ;
#9839=EDGE_CURVE ( 'NONE', #716, #2686, #1684, .T. ) ;
#9841=LINE ( 'NONE', #7521, #713 ) ;
#9843=ORIENTED_EDGE ( 'NONE', *, *, #3926, .T. ) ;
#9845=CARTESIAN_POINT ( 'NONE',  ( -10.35533905932741128, 4.312500000000000888, -24.99999999999996803 ) ) ;
#9849=DIRECTION ( 'NONE',  ( -0.000000000000000000, -1.000000000000000000, -0.000000000000000000 ) ) ;
#9851=CARTESIAN_POINT ( 'NONE',  ( 0.000000000000000000, 20.00000000000000355, 0.000000000000000000 ) ) ;
#9857=EDGE_CURVE ( 'NONE', #1695, #6661, #1461, .T. ) ;
#9861=DIRECTION ( 'NONE',  ( -0.4999999999999887312, 0.000000000000000000, 0.8660254037844451469 ) ) ;
#9865=AXIS2_PLACEMENT_3D ( 'NONE', #9610, #3801, #3693 ) ;
#9867=CARTESIAN_POINT ( 'NONE',  ( -7.276923788646446845, -0.001000000000001000089, 18.60400172474275848 ) ) ;
#9868=CIRCLE ( 'NONE', #3892, 2.999999999999997335 ) ;
#9869=CARTESIAN_POINT ( 'NONE',  ( 24.62111388750000174, 2.456249999044084475, -10.19839929293505776 ) ) ;
#9872=DIRECTION ( 'NONE',  ( 0.000000000000000000, 1.000000000000000000, 0.000000000000000000 ) ) ;
#9874=CARTESIAN_POINT ( 'NONE',  ( 1.507608415688466075E-15, 1.468749999044084431, -24.62111388750000174 ) ) ;
#9876=EDGE_LOOP ( 'NONE', ( #8792, #8406, #3868, #2155 ) ) ;
#9877=ORIENTED_EDGE ( 'NONE', *, *, #4709, .T. ) ;
#9882=CARTESIAN_POINT ( 'NONE',  ( 17.40975659021752620, 5.268749999044085364, 17.40975659021753330 ) ) ;
#9887=FACE_OUTER_BOUND ( 'NONE', #1458, .T. ) ;
#9890=CARTESIAN_POINT ( 'NONE',  ( 25.00000000000000000, 0.6124999980881691286, 0.000000000000000000 ) ) ;
#9891=EDGE_CURVE ( 'NONE', #3964, #7240, #10103, .T. ) ;
#9894=VERTEX_POINT ( 'NONE', #5013 ) ;
#9895=EDGE_LOOP ( 'NONE', ( #1873, #7514, #140, #1538 ) ) ;
#9900=FACE_OUTER_BOUND ( 'NONE', #4408, .T. ) ;
#9901=DIRECTION ( 'NONE',  ( -0.000000000000000000, 1.000000000000000000, -0.000000000000000000 ) ) ;
#9903=AXIS2_PLACEMENT_3D ( 'NONE', #9314, #3400, #5139 ) ;
#9910=ORIENTED_EDGE ( 'NONE', *, *, #1803, .F. ) ;
#9911=VECTOR ( 'NONE', #5122, 1000.000000000000000 ) ;
#9915=FACE_OUTER_BOUND ( 'NONE', #637, .T. ) ;
#9917=CARTESIAN_POINT ( 'NONE',  ( -15.60400172474278158, -0.001000000000001000089, -12.47307621135316680 ) ) ;
#9918=CARTESIAN_POINT ( 'NONE',  ( 0.000000000000000000, 28.00000000000000000, 0.000000000000000000 ) ) ;
#9924=AXIS2_PLACEMENT_3D ( 'NONE', #9918, #6009, #6728 ) ;
#9927=CARTESIAN_POINT ( 'NONE',  ( 17.40975659021752620, 2.268749999044084475, 17.40975659021753330 ) ) ;
#9928=EDGE_LOOP ( 'NONE', ( #6498, #6172, #5202, #10007 ) ) ;
#9934=CARTESIAN_POINT ( 'NONE',  ( 24.62111388749999108, 2.156249999044084653, 10.19839929293507730 ) ) ;
#9936=VECTOR ( 'NONE', #2294, 1000.000000000000000 ) ;
#9938=VERTEX_POINT ( 'NONE', #1737 ) ;
#9941=CARTESIAN_POINT ( 'NONE',  ( 9.874999999999895195, 28.00000000000000000, -17.10400172474272651 ) ) ;
#9942=CARTESIAN_POINT ( 'NONE',  ( -10.19839929293505776, 1.531249999044084653, -24.62111388750000174 ) ) ;
#9943=ORIENTED_EDGE ( 'NONE', *, *, #3539, .F. ) ;
#9948=DIRECTION ( 'NONE',  ( -0.000000000000000000, -1.000000000000000000, -0.000000000000000000 ) ) ;
#9949=DIRECTION ( 'NONE',  ( -0.000000000000000000, -1.000000000000000000, -0.000000000000000000 ) ) ;
#9950=VERTEX_POINT ( 'NONE', #2547 ) ;
#9951=VERTEX_POINT ( 'NONE', #3258 ) ;
#9952=EDGE_CURVE ( 'NONE', #5793, #6120, #6716, .T. ) ;
#9954=CARTESIAN_POINT ( 'NONE',  ( -10.19839929293507552, 3.081249999044084475, 24.62111388749999463 ) ) ;
#9955=CARTESIAN_POINT ( 'NONE',  ( -24.62111388750000174, 0.7187499990440845421, -3.015216831376932151E-15 ) ) ;
#9956=EDGE_CURVE ( 'NONE', #7963, #7237, #2393, .T. ) ;
#9958=EDGE_LOOP ( 'NONE', ( #10555, #1491, #3690, #5772 ) ) ;
#9960=CARTESIAN_POINT ( 'NONE',  ( -5.276923788646495694, 25.00000000000000000, 15.13990010960498012 ) ) ;
#9961=DIRECTION ( 'NONE',  ( 0.000000000000000000, 1.000000000000000000, 0.000000000000000000 ) ) ;
#9971=LINE ( 'NONE', #4231, #9911 ) ;
#9980=FACE_OUTER_BOUND ( 'NONE', #5134, .T. ) ;
#9981=ORIENTED_EDGE ( 'NONE', *, *, #8143, .T. ) ;
#9985=DIRECTION ( 'NONE',  ( -0.000000000000000000, -1.000000000000000000, -0.000000000000000000 ) ) ;
#9986=CARTESIAN_POINT ( 'NONE',  ( -24.62111388750000174, 2.656249999044085097, -10.19839929293506131 ) ) ;
#9988=VERTEX_POINT ( 'NONE', #255 ) ;
#9990=DIRECTION ( 'NONE',  ( 0.000000000000000000, 0.000000000000000000, 1.000000000000000000 ) ) ;
#9991=CARTESIAN_POINT ( 'NONE',  ( 10.19839929293505953, 3.406249999044085097, -24.62111388750000174 ) ) ;
#9992=DIRECTION ( 'NONE',  ( 0.4999999999999977796, 0.000000000000000000, -0.8660254037844399289 ) ) ;
#9998=EDGE_CURVE ( 'NONE', #10484, #7237, #1194, .T. ) ;
#9999=CYLINDRICAL_SURFACE ( 'NONE', #3679, 25.00000000000000000 ) ;
#10000=DIRECTION ( 'NONE',  ( 0.4999999999999947820, 0.000000000000000000, -0.8660254037844417052 ) ) ;
#10001=DIRECTION ( 'NONE',  ( -0.000000000000000000, -1.000000000000000000, -0.000000000000000000 ) ) ;
#10005=ORIENTED_EDGE ( 'NONE', *, *, #5056, .T. ) ;
#10006=ORIENTED_EDGE ( 'NONE', *, *, #7486, .F. ) ;
#10007=ORIENTED_EDGE ( 'NONE', *, *, #9956, .F. ) ;
#10009=CARTESIAN_POINT ( 'NONE',  ( 17.40975659021752975, 0.5187499990440845865, -17.40975659021752975 ) ) ;
#10012=MECHANICAL_DESIGN_GEOMETRIC_PRESENTATION_REPRESENTATION('',(#7728),#1036);
#10018=DIRECTION ( 'NONE',  ( -0.000000000000000000, 1.000000000000000000, -0.000000000000000000 ) ) ;
#10022=ORIENTED_EDGE ( 'NONE', *, *, #439, .T. ) ;
#10025=CARTESIAN_POINT ( 'NONE',  ( 0.000000000000000000, 28.00000000000000000, 0.000000000000000000 ) ) ;
#10032=ORIENTED_EDGE ( 'NONE', *, *, #3014, .F. ) ;
#10037=ORIENTED_EDGE ( 'NONE', *, *, #3833, .F. ) ;
#10038=DIRECTION ( 'NONE',  ( 0.000000000000000000, 0.000000000000000000, 1.000000000000000000 ) ) ;
#10040=LINE ( 'NONE', #4191, #6420 ) ;
#10043=CARTESIAN_POINT ( 'NONE',  ( -10.19839929293507375, 2.906249999044085541, 24.62111388749999108 ) ) ;
#10044=EDGE_LOOP ( 'NONE', ( #6635, #7589, #2031, #3615 ) ) ;
#10048=EDGE_CURVE ( 'NONE', #3835, #6439, #9048, .T. ) ;
#10051=CARTESIAN_POINT ( 'NONE',  ( -17.40975659021753330, 1.843749999044084653, 17.40975659021752975 ) ) ;
#10055=CARTESIAN_POINT ( 'NONE',  ( 25.00000000000000000, 1.674999998088169351, -10.35533905932737753 ) ) ;
#10056=CARTESIAN_POINT ( 'NONE',  ( -5.276923788646812774, 25.00000000000000000, -15.13990010960486821 ) ) ;
#10057=CARTESIAN_POINT ( 'NONE',  ( 0.000000000000000000, 31.00000000000000000, 0.000000000000000000 ) ) ;
#10058=CARTESIAN_POINT ( 'NONE',  ( -7.276923788646446845, -0.001000000000001000089, 18.60400172474275848 ) ) ;
#10064=EDGE_LOOP ( 'NONE', ( #8034, #9296, #1335, #4331 ) ) ;
#10066=CIRCLE ( 'NONE', #7245, 2.999999999999997335 ) ;
#10068=CARTESIAN_POINT ( 'NONE',  ( 1.507608415688466075E-15, 1.643749999044084475, -24.62111388750000174 ) ) ;
#10069=CARTESIAN_POINT ( 'NONE',  ( -10.19839929293507552, 0.9062499990440844311, 24.62111388749999463 ) ) ;
#10070=DIRECTION ( 'NONE',  ( 0.000000000000000000, 1.000000000000000000, 0.000000000000000000 ) ) ;
#10077=ORIENTED_EDGE ( 'NONE', *, *, #335, .F. ) ;
#10079=ORIENTED_EDGE ( 'NONE', *, *, #1715, .F. ) ;
#10086=EDGE_CURVE ( 'NONE', #5017, #3638, #976, .T. ) ;
#10089=CARTESIAN_POINT ( 'NONE',  ( 25.00000000000000000, 5.000000000000000000, 0.000000000000000000 ) ) ;
#10091=DIRECTION ( 'NONE',  ( -0.000000000000000000, -1.000000000000000000, -0.000000000000000000 ) ) ;
#10092=ADVANCED_FACE ( 'NONE', ( #6171 ), #3612, .F. ) ;
#10096=VECTOR ( 'NONE', #7835, 1000.000000000000000 ) ;
#10097=DIRECTION ( 'NONE',  ( 3.708321773340234242E-15, 0.000000000000000000, 1.000000000000000000 ) ) ;
#10101=CARTESIAN_POINT ( 'NONE',  ( -25.00000000000001066, 5.174999998088170017, 10.35533905932737397 ) ) ;
#10103=CIRCLE ( 'NONE', #3383, 25.00000000000000000 ) ;
#10105=VERTEX_POINT ( 'NONE', #3605 ) ;
#10107=ORIENTED_EDGE ( 'NONE', *, *, #6080, .F. ) ;
#10114=DIRECTION ( 'NONE',  ( -0.000000000000000000, -1.000000000000000000, -0.000000000000000000 ) ) ;
#10115=DIRECTION ( 'NONE',  ( 0.000000000000000000, 0.000000000000000000, -1.000000000000000000 ) ) ;
#10118=DIRECTION ( 'NONE',  ( 0.000000000000000000, 1.000000000000000000, 0.000000000000000000 ) ) ;
#10121=AXIS2_PLACEMENT_3D ( 'NONE', #9917, #2353, #6406 ) ;
#10123=ORIENTED_EDGE ( 'NONE', *, *, #247, .T. ) ;
#10126=DIRECTION ( 'NONE',  ( 0.000000000000000000, 0.000000000000000000, -1.000000000000000000 ) ) ;
#10128=CARTESIAN_POINT ( 'NONE',  ( 24.62111388750000174, 0.4562499990440845310, -10.19839929293505776 ) ) ;
#10129=CARTESIAN_POINT ( 'NONE',  ( -25.00000000000001421, 0.5625000000000001110, 10.35533905932737397 ) ) ;
#10131=VERTEX_POINT ( 'NONE', #5282 ) ;
#10156=DIRECTION ( 'NONE',  ( 0.000000000000000000, 0.000000000000000000, -1.000000000000000000 ) ) ;
#10158=EDGE_CURVE ( 'NONE', #8118, #5055, #6059, .T. ) ;
#10170=CARTESIAN_POINT ( 'NONE',  ( 19.75000000000001066, 25.00000000000000000, 2.999999999999927613 ) ) ;
#10174=DIRECTION ( 'NONE',  ( 0.000000000000000000, 0.000000000000000000, 1.000000000000000000 ) ) ;
#10177=CARTESIAN_POINT ( 'NONE',  ( 19.74999999999998934, 25.00000000000000000, -3.000000000000067946 ) ) ;
#10178=CARTESIAN_POINT ( 'NONE',  ( -10.19839929293505776, 0.7062499990440844755, -24.62111388750000174 ) ) ;
#10179=CARTESIAN_POINT ( 'NONE',  ( -17.40975659021752975, 2.593749999044084653, -17.40975659021752975 ) ) ;
#10180=CARTESIAN_POINT ( 'NONE',  ( -12.47307621135344391, -0.001000000000001000089, -15.60400172474256131 ) ) ;
#10183=CARTESIAN_POINT ( 'NONE',  ( 12.47307621135333200, 28.00000000000000000, 15.60400172474264835 ) ) ;
#10185=LINE ( 'NONE', #1970, #4970 ) ;
#10189=VERTEX_POINT ( 'NONE', #4455 ) ;
#10190=ORIENTED_EDGE ( 'NONE', *, *, #5575, .T. ) ;
#10195=DIRECTION ( 'NONE',  ( 0.000000000000000000, 1.000000000000000000, 0.000000000000000000 ) ) ;
#10201=AXIS2_PLACEMENT_3D ( 'NONE', #1850, #3490, #5233 ) ;
#10204=LINE ( 'NONE', #2619, #4583 ) ;
#10207=FACE_OUTER_BOUND ( 'NONE', #7993, .T. ) ;
#10208=CYLINDRICAL_SURFACE ( 'NONE', #9903, 2.999999999999999112 ) ;
#10212=CYLINDRICAL_SURFACE ( 'NONE', #497, 25.00000000000000000 ) ;
#10214=LINE ( 'NONE', #5859, #190 ) ;
#10219=CARTESIAN_POINT ( 'NONE',  ( -17.67766952966368876, 0.9874999980881691286, -17.67766952966369232 ) ) ;
#10222=FACE_BOUND ( 'NONE', #2816, .T. ) ;
#10223=EDGE_CURVE ( 'NONE', #2972, #5481, #905, .T. ) ;
#10230=EDGE_LOOP ( 'NONE', ( #4202, #5687, #3260, #1566 ) ) ;
#10232=EDGE_CURVE ( 'NONE', #2102, #4070, #4859, .T. ) ;
#10233=CARTESIAN_POINT ( 'NONE',  ( 9.875000000000023093, 25.00000000000000000, 17.10400172474264835 ) ) ;
#10235=CARTESIAN_POINT ( 'NONE',  ( 1.530808498934191521E-15, 0.8624999980881691286, -25.00000000000000000 ) ) ;
#10236=CARTESIAN_POINT ( 'NONE',  ( 10.35533905932738286, 4.424999998088169129, 24.99999999999999645 ) ) ;
#10237=CARTESIAN_POINT ( 'NONE',  ( -17.40975659021752975, 4.593749999044084653, -17.40975659021752975 ) ) ;
#10238=CARTESIAN_POINT ( 'NONE',  ( -25.00000000000000000, 3.049999998088169129, -10.35533905932738108 ) ) ;
#10239=CIRCLE ( 'NONE', #3526, 25.00000000000000000 ) ;
#10240=EDGE_CURVE ( 'NONE', #3898, #1513, #6820, .T. ) ;
#10244=CARTESIAN_POINT ( 'NONE',  ( -7.276923788646446845, 28.00000000000000000, 18.60400172474275848 ) ) ;
#10247=EDGE_LOOP ( 'NONE', ( #9463, #9104, #7183, #6704, #9425 ) ) ;
#10249=ADVANCED_FACE ( 'NONE', ( #9283 ), #6345, .F. ) ;
#10250=VECTOR ( 'NONE', #4160, 1000.000000000000000 ) ;
#10252=ORIENTED_EDGE ( 'NONE', *, *, #8344, .T. ) ;
#10259=CARTESIAN_POINT ( 'NONE',  ( -25.00000000000000000, 1.437500000000000000, -10.35533905932738108 ) ) ;
#10260=CARTESIAN_POINT ( 'NONE',  ( 17.40975659021752975, 4.518749999044084475, -17.40975659021752975 ) ) ;
#10273=CARTESIAN_POINT ( 'NONE',  ( 17.40975659021752620, 5.093749999044084653, 17.40975659021753330 ) ) ;
#10281=CARTESIAN_POINT ( 'NONE',  ( 24.62111388749999463, 4.156249999044083765, 10.19839929293507730 ) ) ;
#10282=CARTESIAN_POINT ( 'NONE',  ( -10.19839929293505776, 1.706249999044084698, -24.62111388750000174 ) ) ;
#10284=PLANE ( 'NONE',  #7940 ) ;
#10286=CARTESIAN_POINT ( 'NONE',  ( 25.00000000000000000, 1.612499998088169351, 0.000000000000000000 ) ) ;
#10287=VECTOR ( 'NONE', #1310, 1000.000000000000000 ) ;
#10288=FACE_BOUND ( 'NONE', #6549, .T. ) ;
#10294=ORIENTED_EDGE ( 'NONE', *, *, #2650, .F. ) ;
#10298=CARTESIAN_POINT ( 'NONE',  ( -10.19839929293507552, 1.081249999044084475, 24.62111388749999463 ) ) ;
#10299=CARTESIAN_POINT ( 'NONE',  ( -25.00000000000000000, 4.049999998088169129, -10.35533905932738108 ) ) ;
#10300=AXIS2_PLACEMENT_3D ( 'NONE', #1215, #1170, #2741 ) ;
#10301=CARTESIAN_POINT ( 'NONE',  ( 10.19839929293506486, 3.031249999044084653, 24.62111388749999819 ) ) ;
#10306=DIRECTION ( 'NONE',  ( -0.000000000000000000, -1.000000000000000000, -0.000000000000000000 ) ) ;
#10312=VERTEX_POINT ( 'NONE', #4504 ) ;
#10315=CARTESIAN_POINT ( 'NONE',  ( -3.000000000000000888, -0.001000000000001000089, -15.75000000000000355 ) ) ;
#10321=CARTESIAN_POINT ( 'NONE',  ( -7.276923788646447733, 25.00000000000000000, 18.60400172474275848 ) ) ;
#10323=CARTESIAN_POINT ( 'NONE',  ( -4.522825247065398226E-15, 5.143749999044084475, 24.62111388750000174 ) ) ;
#10324=EDGE_CURVE ( 'NONE', #3699, #3734, #4258, .T. ) ;
#10327=CARTESIAN_POINT ( 'NONE',  ( -18.60400172474273717, 28.00000000000000000, -7.276923788646511682 ) ) ;
#10329=DIRECTION ( 'NONE',  ( 0.000000000000000000, 0.000000000000000000, 1.000000000000000000 ) ) ;
#10334=CARTESIAN_POINT ( 'NONE',  ( -17.40975659021752975, 4.593749999044084653, -17.40975659021752975 ) ) ;
#10343=CARTESIAN_POINT ( 'NONE',  ( -4.592425496802574367E-15, 4.750000000000000000, 25.00000000000000000 ) ) ;
#10345=CARTESIAN_POINT ( 'NONE',  ( -10.35533905932739174, 2.299999998088169129, 24.99999999999999289 ) ) ;
#10346=ORIENTED_EDGE ( 'NONE', *, *, #9998, .F. ) ;
#10350=CARTESIAN_POINT ( 'NONE',  ( -10.35533905932739174, 2.299999998088168685, 24.99999999999999289 ) ) ;
#10351=CARTESIAN_POINT ( 'NONE',  ( -24.62111388750000174, 3.656249999044084653, -10.19839929293506131 ) ) ;
#10353=DIRECTION ( 'NONE',  ( -0.000000000000000000, -1.000000000000000000, -0.000000000000000000 ) ) ;
#10354=FACE_BOUND ( 'NONE', #607, .T. ) ;
#10358=ORIENTED_EDGE ( 'NONE', *, *, #5846, .T. ) ;
#10359=VERTEX_POINT ( 'NONE', #6031 ) ;
#10360=EDGE_LOOP ( 'NONE', ( #9536, #2056, #4067, #5642, #6060 ) ) ;
#10363=DIRECTION ( 'NONE',  ( 0.8660254037844362651, 0.000000000000000000, -0.5000000000000041078 ) ) ;
#10367=( BOUNDED_CURVE ( )  B_SPLINE_CURVE ( 2, ( #3012, #7031, #2860, #6205, #9563, #5380, #6258, #5468, #8835 ),
 .UNSPECIFIED., .F., .F. ) 
 B_SPLINE_CURVE_WITH_KNOTS ( ( 3, 2, 2, 2, 3 ),
 ( 0.05000000000000000278, 0.07500000000000001110, 0.1000000000000000194, 0.1250000000000000278, 0.1500000000000000222 ),
 .UNSPECIFIED. ) 
 CURVE ( )  GEOMETRIC_REPRESENTATION_ITEM ( )  RATIONAL_B_SPLINE_CURVE ( ( 1.000000000000000000, 0.9238795325112867385, 1.000000000000000000, 0.9238795325112867385, 1.000000000000000000, 0.9238795325112867385, 1.000000000000000000, 0.9238795325112866275, 1.000000000000000000 ) ) 
 REPRESENTATION_ITEM ( '' )  );
#10368=DIRECTION ( 'NONE',  ( 0.000000000000000000, 0.000000000000000000, 1.000000000000000000 ) ) ;
#10369=EDGE_CURVE ( 'NONE', #5054, #2200, #2164, .T. ) ;
#10370=DIRECTION ( 'NONE',  ( 0.000000000000000000, 1.000000000000000000, 0.000000000000000000 ) ) ;
#10371=DIRECTION ( 'NONE',  ( 0.000000000000000000, 0.000000000000000000, -1.000000000000000000 ) ) ;
#10372=CARTESIAN_POINT ( 'NONE',  ( -24.62111388750000884, 3.956249999044084920, 10.19839929293505421 ) ) ;
#10373=VERTEX_POINT ( 'NONE', #1324 ) ;
#10377=EDGE_LOOP ( 'NONE', ( #4578, #8977, #8035, #65 ) ) ;
#10378=CARTESIAN_POINT ( 'NONE',  ( -17.10400172474275848, 25.00000000000000000, -9.874999999999836575 ) ) ;
#10379=CARTESIAN_POINT ( 'NONE',  ( 15.60400172474260927, 25.00000000000000000, -12.47307621135339062 ) ) ;
#10382=DIRECTION ( 'NONE',  ( -0.000000000000000000, -1.000000000000000000, -0.000000000000000000 ) ) ;
#10383=CARTESIAN_POINT ( 'NONE',  ( 13.63990010960492860, -0.001000000000001000089, 7.874999999999965361 ) ) ;
#10387=VECTOR ( 'NONE', #5146, 1000.000000000000000 ) ;
#10389=CARTESIAN_POINT ( 'NONE',  ( 1.530808498934191521E-15, 2.250000000000000444, -25.00000000000000000 ) ) ;
#10391=CYLINDRICAL_SURFACE ( 'NONE', #7910, 2.999999999999997335 ) ;
#10392=CARTESIAN_POINT ( 'NONE',  ( 17.40975659021752620, 1.268749999044084475, 17.40975659021753330 ) ) ;
#10393=ORIENTED_EDGE ( 'NONE', *, *, #9160, .F. ) ;
#10394=CARTESIAN_POINT ( 'NONE',  ( 3.061616997868383043E-15, 20.00000000000000355, 25.00000000000000000 ) ) ;
#10395=CARTESIAN_POINT ( 'NONE',  ( 0.000000000000000000, 20.00000000000000355, -25.00000000000000000 ) ) ;
#10397=LINE ( 'NONE', #2011, #5775 ) ;
#10398=VERTEX_POINT ( 'NONE', #441 ) ;
#10399=ADVANCED_FACE ( 'NONE', ( #6303 ), #10391, .F. ) ;
#10404=CARTESIAN_POINT ( 'NONE',  ( -4.592425496802574367E-15, 3.362499998088169129, 25.00000000000000000 ) ) ;
#10405=CARTESIAN_POINT ( 'NONE',  ( 25.00000000000000000, 5.000000000000000000, 0.000000000000000000 ) ) ;
#10409=FACE_OUTER_BOUND ( 'NONE', #2677, .T. ) ;
#10410=CIRCLE ( 'NONE', #6356, 2.999999999999997335 ) ;
#10419=DIRECTION ( 'NONE',  ( -0.8660254037844431485, 0.000000000000000000, -0.4999999999999920064 ) ) ;
#10422=DIRECTION ( 'NONE',  ( 0.000000000000000000, 0.000000000000000000, -1.000000000000000000 ) ) ;
#10424=CARTESIAN_POINT ( 'NONE',  ( -17.67766952966369232, 1.625000000000000222, 17.67766952966368876 ) ) ;
#10425=CARTESIAN_POINT ( 'NONE',  ( -4.522825247065398226E-15, 4.143749999044083587, 24.62111388750000174 ) ) ;
#10430=EDGE_CURVE ( 'NONE', #3638, #5087, #8782, .T. ) ;
#10436=DIRECTION ( 'NONE',  ( -1.734723475976808672E-15, 0.000000000000000000, 1.000000000000000000 ) ) ;
#10447=ORIENTED_EDGE ( 'NONE', *, *, #916, .T. ) ;
#10452=EDGE_CURVE ( 'NONE', #1429, #6472, #10367, .T. ) ;
#10460=DIRECTION ( 'NONE',  ( 0.000000000000000000, 0.000000000000000000, 1.000000000000000000 ) ) ;
#10462=AXIS2_PLACEMENT_3D ( 'NONE', #8812, #7013, #10371 ) ;
#10463=CARTESIAN_POINT ( 'NONE',  ( 10.19839929293506486, 1.206249999044084698, 24.62111388749999819 ) ) ;
#10464=CARTESIAN_POINT ( 'NONE',  ( -25.00000000000001421, 2.562500000000000444, 10.35533905932737397 ) ) ;
#10467=DIRECTION ( 'NONE',  ( 0.000000000000000000, 0.000000000000000000, 1.000000000000000000 ) ) ;
#10471=EDGE_CURVE ( 'NONE', #4838, #2806, #9662, .T. ) ;
#10472=AXIS2_PLACEMENT_3D ( 'NONE', #9477, #3671, #1152 ) ;
#10473=EDGE_LOOP ( 'NONE', ( #3907, #10732, #6185, #679 ) ) ;
#10480=CARTESIAN_POINT ( 'NONE',  ( 0.000000000000000000, 20.00000000000000355, 0.000000000000000000 ) ) ;
#10484=VERTEX_POINT ( 'NONE', #5685 ) ;
#10485=EDGE_LOOP ( 'NONE', ( #2221, #4719, #10792, #584 ) ) ;
#10486=VECTOR ( 'NONE', #1692, 1000.000000000000000 ) ;
#10489=CYLINDRICAL_SURFACE ( 'NONE', #700, 2.999999999999997335 ) ;
#10491=CARTESIAN_POINT ( 'NONE',  ( -17.10400172474254532, -0.001000000000001000089, 12.87500000000020073 ) ) ;
#10492=LINE ( 'NONE', #7688, #2140 ) ;
#10495=( BOUNDED_CURVE ( )  B_SPLINE_CURVE ( 2, ( #288, #3652, #235, #9516, #5326, #3596, #6984, #7035, #8016 ),
 .UNSPECIFIED., .F., .F. ) 
 B_SPLINE_CURVE_WITH_KNOTS ( ( 3, 2, 2, 2, 3 ),
 ( 0.4500000000000000111, 0.4749999999999999778, 0.5000000000000000000, 0.5250000000000000222, 0.5500000000000000444 ),
 .UNSPECIFIED. ) 
 CURVE ( )  GEOMETRIC_REPRESENTATION_ITEM ( )  RATIONAL_B_SPLINE_CURVE ( ( 1.000000000000000000, 0.9238795325112867385, 1.000000000000000000, 0.9238795325112867385, 1.000000000000000000, 0.9238795325112867385, 1.000000000000000000, 0.9238795325112867385, 1.000000000000000000 ) ) 
 REPRESENTATION_ITEM ( '' )  );
#10497=CARTESIAN_POINT ( 'NONE',  ( 1.530808498934191521E-15, 3.250000000000000444, -25.00000000000000000 ) ) ;
#10498=CARTESIAN_POINT ( 'NONE',  ( -4.522825247065398226E-15, 1.143749999044084475, 24.62111388750000174 ) ) ;
#10504=CARTESIAN_POINT ( 'NONE',  ( 25.00000000000000000, 2.674999998088169573, -10.35533905932737753 ) ) ;
#10508=ORIENTED_EDGE ( 'NONE', *, *, #6647, .T. ) ;
#10512=EDGE_CURVE ( 'NONE', #1695, #8288, #1580, .T. ) ;
#10515=CARTESIAN_POINT ( 'NONE',  ( -24.62111388750000884, 2.956249999044084475, 10.19839929293505421 ) ) ;
#10516=CARTESIAN_POINT ( 'NONE',  ( -10.35533905932737575, 1.312500000000000444, -25.00000000000000000 ) ) ;
#10518=CARTESIAN_POINT ( 'NONE',  ( 12.47307621135333200, 25.00000000000000000, 15.60400172474264835 ) ) ;
#10520=CARTESIAN_POINT ( 'NONE',  ( 1.530808498934191521E-15, 3.862499998088169573, -25.00000000000000000 ) ) ;
#10527=DIRECTION ( 'NONE',  ( 0.000000000000000000, 0.000000000000000000, 1.000000000000000000 ) ) ;
#10528=PLANE ( 'NONE',  #3005 ) ;
#10546=CARTESIAN_POINT ( 'NONE',  ( -9.875000000000143885, -0.001000000000001000089, -17.10400172474258085 ) ) ;
#10547=CARTESIAN_POINT ( 'NONE',  ( -24.62111388750000174, 4.893749999044084475, -3.015216831376932151E-15 ) ) ;
#10549=CARTESIAN_POINT ( 'NONE',  ( 24.81055694375000087, 0.1093749995220422710, 0.000000000000000000 ) ) ;
#10554=CYLINDRICAL_SURFACE ( 'NONE', #331, 2.999999999999999112 ) ;
#10555=ORIENTED_EDGE ( 'NONE', *, *, #1979, .T. ) ;
#10556=ORIENTED_EDGE ( 'NONE', *, *, #130, .T. ) ;
#10561=CARTESIAN_POINT ( 'NONE',  ( 24.62111388750000174, 4.393749999044085364, 0.000000000000000000 ) ) ;
#10563=CARTESIAN_POINT ( 'NONE',  ( 10.35533905932738286, 1.812500000000000222, 24.99999999999999645 ) ) ;
#10565=DIRECTION ( 'NONE',  ( -0.8660254037844431485, 0.000000000000000000, -0.4999999999999922839 ) ) ;
#10567=DIRECTION ( 'NONE',  ( 2.168404344971010594E-16, -0.000000000000000000, 1.000000000000000000 ) ) ;
#10568=CARTESIAN_POINT ( 'NONE',  ( 24.99999999999999289, 0.9375000000000000000, 10.35533905932739529 ) ) ;
#10570=ADVANCED_FACE ( 'NONE', ( #10207 ), #2621, .F. ) ;
#10573=UNCERTAINTY_MEASURE_WITH_UNIT (LENGTH_MEASURE( 1.000000000000000082E-05 ), #4787, 'distance_accuracy_value', 'NONE');
#10579=DIRECTION ( 'NONE',  ( -0.000000000000000000, -1.000000000000000000, -0.000000000000000000 ) ) ;
#10580=DIRECTION ( 'NONE',  ( -0.8660254037844417052, 0.000000000000000000, -0.4999999999999947820 ) ) ;
#10584=AXIS2_PLACEMENT_3D ( 'NONE', #1878, #8550, #998 ) ;
#10585=VECTOR ( 'NONE', #3372, 999.9999999999998863 ) ;
#10594=CARTESIAN_POINT ( 'NONE',  ( 0.000000000000000000, 28.00000000000000000, 0.000000000000000000 ) ) ;
#10595=EDGE_CURVE ( 'NONE', #10398, #3501, #5777, .T. ) ;
#10596=VERTEX_POINT ( 'NONE', #2684 ) ;
#10602=CARTESIAN_POINT ( 'NONE',  ( 24.62111388749999108, 5.331249999044085364, 10.19839929293507730 ) ) ;
#10614=CARTESIAN_POINT ( 'NONE',  ( -24.62111388750000174, 1.831249999044084475, -10.19839929293506131 ) ) ;
#10615=ORIENTED_EDGE ( 'NONE', *, *, #9343, .F. ) ;
#10616=CARTESIAN_POINT ( 'NONE',  ( 10.35533905932737930, 4.187500000000000000, -25.00000000000000000 ) ) ;
#10617=( NAMED_UNIT ( * ) PLANE_ANGLE_UNIT ( ) SI_UNIT ( $, .RADIAN. ) );
#10619=DIRECTION ( 'NONE',  ( 0.000000000000000000, 0.000000000000000000, 1.000000000000000000 ) ) ;
#10625=ORIENTED_EDGE ( 'NONE', *, *, #7281, .T. ) ;
#10626=CIRCLE ( 'NONE', #2331, 2.999999999999997335 ) ;
#10628=AXIS2_PLACEMENT_3D ( 'NONE', #3443, #3564, #10419 ) ;
#10629=DIRECTION ( 'NONE',  ( 0.000000000000000000, 1.000000000000000000, 0.000000000000000000 ) ) ;
#10633=ORIENTED_EDGE ( 'NONE', *, *, #7656, .T. ) ;
#10634=DIRECTION ( 'NONE',  ( -0.000000000000000000, -1.000000000000000000, -0.000000000000000000 ) ) ;
#10639=EDGE_CURVE ( 'NONE', #10668, #3974, #8950, .T. ) ;
#10640=EDGE_CURVE ( 'NONE', #8568, #9592, #8042, .T. ) ;
#10642=VERTEX_POINT ( 'NONE', #10327 ) ;
#10646=ADVANCED_FACE ( 'NONE', ( #2739 ), #822, .F. ) ;
#10648=AXIS2_PLACEMENT_3D ( 'NONE', #8879, #3853, #1314 ) ;
#10650=CARTESIAN_POINT ( 'NONE',  ( 24.99999999999999289, 4.549999998088169129, 10.35533905932739529 ) ) ;
#10658=CARTESIAN_POINT ( 'NONE',  ( -12.13990010960501031, 28.00000000000000000, -10.47307621135320410 ) ) ;
#10660=CARTESIAN_POINT ( 'NONE',  ( -17.40975659021753330, 2.018749999044084475, 17.40975659021752975 ) ) ;
#10661=EDGE_LOOP ( 'NONE', ( #7930, #2312, #84, #3409 ) ) ;
#10664=CARTESIAN_POINT ( 'NONE',  ( 7.347880794884118750E-16, 28.00000000000000000, 5.999999999999999112 ) ) ;
#10665=ORIENTED_EDGE ( 'NONE', *, *, #6940, .T. ) ;
#10667=CARTESIAN_POINT ( 'NONE',  ( -10.19839929293507375, 0.9062499990440844311, 24.62111388749999108 ) ) ;
#10668=VERTEX_POINT ( 'NONE', #10379 ) ;
#10672=CARTESIAN_POINT ( 'NONE',  ( -24.62111388750000174, 2.893749999044084475, -3.015216831376932151E-15 ) ) ;
#10673=VERTEX_POINT ( 'NONE', #7072 ) ;
#10676=CARTESIAN_POINT ( 'NONE',  ( -7.276923788646840308, 28.00000000000000000, -18.60400172474260216 ) ) ;
#10681=ORIENTED_EDGE ( 'NONE', *, *, #6350, .F. ) ;
#10682=ORIENTED_EDGE ( 'NONE', *, *, #2321, .F. ) ;
#10685=CARTESIAN_POINT ( 'NONE',  ( -17.67766952966368876, 4.375000000000000000, -17.67766952966369232 ) ) ;
#10689=CARTESIAN_POINT ( 'NONE',  ( -7.276923788646448621, 28.00000000000000000, 18.60400172474275848 ) ) ;
#10692=ORIENTED_EDGE ( 'NONE', *, *, #5831, .T. ) ;
#10695=CARTESIAN_POINT ( 'NONE',  ( -18.60400172474257730, 28.00000000000000000, 7.276923788646904256 ) ) ;
#10700=EDGE_CURVE ( 'NONE', #2786, #634, #7850, .T. ) ;
#10703=DIRECTION ( 'NONE',  ( 0.8660254037844361541, 0.000000000000000000, -0.5000000000000042188 ) ) ;
#10705=CARTESIAN_POINT ( 'NONE',  ( 10.19839929293506486, 2.206249999044084920, 24.62111388749999819 ) ) ;
#10710=DIRECTION ( 'NONE',  ( 0.000000000000000000, 1.000000000000000000, 0.000000000000000000 ) ) ;
#10712=CARTESIAN_POINT ( 'NONE',  ( 17.40975659021752975, 1.343749999044084653, -17.40975659021752975 ) ) ;
#10719=CARTESIAN_POINT ( 'NONE',  ( -17.40975659021752975, 3.593749999044084653, -17.40975659021752975 ) ) ;
#10721=CARTESIAN_POINT ( 'NONE',  ( 1.530808498934191521E-15, 3.250000000000000444, -25.00000000000000000 ) ) ;
#10723=DIRECTION ( 'NONE',  ( 0.000000000000000000, 0.000000000000000000, 1.000000000000000000 ) ) ;
#10724=CARTESIAN_POINT ( 'NONE',  ( -17.67766952966368876, 1.987499998088169129, -17.67766952966369232 ) ) ;
#10729=CIRCLE ( 'NONE', #6859, 2.999999999999996891 ) ;
#10732=ORIENTED_EDGE ( 'NONE', *, *, #9019, .T. ) ;
#10733=MANIFOLD_SOLID_BREP ( 'Revolve1', #138 ) ;
#10738=LINE ( 'NONE', #2229, #6735 ) ;
#10741=VERTEX_POINT ( 'NONE', #5665 ) ;
#10744=CARTESIAN_POINT ( 'NONE',  ( -18.60400172474273361, 28.00000000000000000, -7.276923788646511682 ) ) ;
#10745=LINE ( 'NONE', #2352, #7290 ) ;
#10750=CIRCLE ( 'NONE', #6004, 2.999999999999999112 ) ;
#10754=ORIENTED_EDGE ( 'NONE', *, *, #8538, .T. ) ;
#10760=CARTESIAN_POINT ( 'NONE',  ( 24.62111388750000174, 4.393749999044084475, 0.000000000000000000 ) ) ;
#10767=CARTESIAN_POINT ( 'NONE',  ( -10.19839929293505776, 1.531249999044084653, -24.62111388750000174 ) ) ;
#10771=EDGE_CURVE ( 'NONE', #2468, #7097, #518, .T. ) ;
#10776=CYLINDRICAL_SURFACE ( 'NONE', #9539, 2.999999999999997335 ) ;
#10777=CARTESIAN_POINT ( 'NONE',  ( 17.40975659021752620, 1.093749999044084653, 17.40975659021753330 ) ) ;
#10778=ORIENTED_EDGE ( 'NONE', *, *, #4227, .T. ) ;
#10779=DIRECTION ( 'NONE',  ( 0.000000000000000000, 1.000000000000000000, 0.000000000000000000 ) ) ;
#10783=FACE_OUTER_BOUND ( 'NONE', #10064, .T. ) ;
#10792=ORIENTED_EDGE ( 'NONE', *, *, #994, .F. ) ;
#10801=DIRECTION ( 'NONE',  ( 0.000000000000000000, 1.000000000000000000, 0.000000000000000000 ) ) ;
#10803=DIRECTION ( 'NONE',  ( 0.000000000000000000, 0.000000000000000000, 1.000000000000000000 ) ) ;
#10804=CIRCLE ( 'NONE', #8692, 2.999999999999997780 ) ;
#10805=ORIENTED_EDGE ( 'NONE', *, *, #8713, .F. ) ;
#10806=VERTEX_POINT ( 'NONE', #11 ) ;
#10808=ORIENTED_EDGE ( 'NONE', *, *, #3331, .T. ) ;
#10810=VECTOR ( 'NONE', #10860, 1000.000000000000000 ) ;
#10814=CARTESIAN_POINT ( 'NONE',  ( 17.67766952966369232, 4.125000000000000000, -17.67766952966369232 ) ) ;
#10819=ORIENTED_EDGE ( 'NONE', *, *, #792, .T. ) ;
#10821=AXIS2_PLACEMENT_3D ( 'NONE', #3569, #9194, #10368 ) ;
#10823=DIRECTION ( 'NONE',  ( -0.000000000000000000, 1.000000000000000000, -0.000000000000000000 ) ) ;
#10825=DIRECTION ( 'NONE',  ( -0.000000000000000000, -1.000000000000000000, -0.000000000000000000 ) ) ;
#10827=CARTESIAN_POINT ( 'NONE',  ( 0.000000000000000000, 31.00000000000000000, 0.000000000000000000 ) ) ;
#10834=CARTESIAN_POINT ( 'NONE',  ( 1.507608415688466075E-15, 1.468749999044084431, -24.62111388750000174 ) ) ;
#10835=DIRECTION ( 'NONE',  ( -0.8660254037844399289, 0.000000000000000000, -0.4999999999999977796 ) ) ;
#10836=EDGE_LOOP ( 'NONE', ( #5703, #1913, #4128, #3980 ) ) ;
#10842=CARTESIAN_POINT ( 'NONE',  ( -9.875000000000143885, 28.00000000000000000, -17.10400172474258085 ) ) ;
#10843=LINE ( 'NONE', #1780, #1575 ) ;
#10844=EDGE_CURVE ( 'NONE', #7005, #10105, #4276, .T. ) ;
#10846=VERTEX_POINT ( 'NONE', #1559 ) ;
#10847=ORIENTED_EDGE ( 'NONE', *, *, #1066, .F. ) ;
#10849=ORIENTED_EDGE ( 'NONE', *, *, #66, .F. ) ;
#10851=CARTESIAN_POINT ( 'NONE',  ( -17.40975659021752975, 0.7687499990440845865, -17.40975659021752975 ) ) ;
#10852=CARTESIAN_POINT ( 'NONE',  ( -10.19839929293505776, 1.531249999044084653, -24.62111388750000174 ) ) ;
#10854=ORIENTED_EDGE ( 'NONE', *, *, #1696, .F. ) ;
#10855=EDGE_CURVE ( 'NONE', #1858, #500, #5617, .T. ) ;
#10857=DIRECTION ( 'NONE',  ( 0.000000000000000000, 1.000000000000000000, 0.000000000000000000 ) ) ;
#10860=DIRECTION ( 'NONE',  ( -1.000000000000000000, 0.000000000000000000, 1.069128445102650095E-14 ) ) ;
#10862=ORIENTED_EDGE ( 'NONE', *, *, #436, .T. ) ;
#10872=CARTESIAN_POINT ( 'NONE',  ( 25.00000000000000000, 0.06249999999999997224, -10.35533905932737753 ) ) ;
#10874=EDGE_CURVE ( 'NONE', #5240, #1695, #6710, .T. ) ;
#10876=DIRECTION ( 'NONE',  ( -0.000000000000000000, 1.000000000000000000, 0.000000000000000000 ) ) ;
#10878=DIRECTION ( 'NONE',  ( -0.000000000000000000, 1.000000000000000000, -0.000000000000000000 ) ) ;
#10882=LINE ( 'NONE', #5084, #7456 ) ;
#10884=CARTESIAN_POINT ( 'NONE',  ( 10.19839929293505953, 2.406249999044085541, -24.62111388750000174 ) ) ;
#10885=ORIENTED_EDGE ( 'NONE', *, *, #7900, .T. ) ;
#10888=CARTESIAN_POINT ( 'NONE',  ( -13.63990010960498367, -0.001000000000001000089, -7.874999999999870326 ) ) ;
#10890=CARTESIAN_POINT ( 'NONE',  ( -17.40975659021753330, 2.843749999044085097, 17.40975659021752975 ) ) ;
#10893=DIRECTION ( 'NONE',  ( 0.000000000000000000, 0.000000000000000000, 1.000000000000000000 ) ) ;
#10897=DIRECTION ( 'NONE',  ( -0.000000000000000000, -1.000000000000000000, -0.000000000000000000 ) ) ;
#10898=CARTESIAN_POINT ( 'NONE',  ( 7.276923788646575630, 25.00000000000000000, -18.60400172474270519 ) ) ;
#10899=ORIENTED_EDGE ( 'NONE', *, *, #3962, .F. ) ;
#10902=ORIENTED_EDGE ( 'NONE', *, *, #2932, .F. ) ;
#10903=ORIENTED_EDGE ( 'NONE', *, *, #10471, .T. ) ;
#10904=EDGE_CURVE ( 'NONE', #7447, #8872, #8633, .T. ) ;
#10905=CARTESIAN_POINT ( 'NONE',  ( -24.62111388750000174, 0.8312499990440843645, -10.19839929293506131 ) ) ;
#10906=CARTESIAN_POINT ( 'NONE',  ( -17.40975659021752975, 1.593749999044084431, -17.40975659021752975 ) ) ;
#10908=EDGE_LOOP ( 'NONE', ( #1503, #9086, #8249, #3820 ) ) ;
#10918=ADVANCED_FACE ( 'NONE', ( #5992 ), #300, .F. ) ;
#10924=EDGE_CURVE ( 'NONE', #652, #93, #139, .T. ) ;
#10925=CARTESIAN_POINT ( 'NONE',  ( 12.13990010960486288, 25.00000000000000000, -10.47307621135337108 ) ) ;
#10926=LINE ( 'NONE', #7544, #1831 ) ;
#10928=ADVANCED_FACE ( 'NONE', ( #188, #2024 ), #3548, .F. ) ;
#10931=CARTESIAN_POINT ( 'NONE',  ( 0.000000000000000000, 28.00000000000000000, 0.000000000000000000 ) ) ;
#10933=ORIENTED_EDGE ( 'NONE', *, *, #8153, .F. ) ;
#10934=CARTESIAN_POINT ( 'NONE',  ( -9.875000000000143885, 25.00000000000000000, -17.10400172474258085 ) ) ;
#10941=CARTESIAN_POINT ( 'NONE',  ( -10.19839929293507375, 3.906249999044085097, 24.62111388749999108 ) ) ;
#10942=ORIENTED_EDGE ( 'NONE', *, *, #9089, .T. ) ;
#10945=EDGE_CURVE ( 'NONE', #1513, #1422, #2598, .T. ) ;
#10946=CARTESIAN_POINT ( 'NONE',  ( 0.000000000000000000, 31.00000000000000000, -7.500000000000000888 ) ) ;
ENDSEC;
END-ISO-10303-21;
